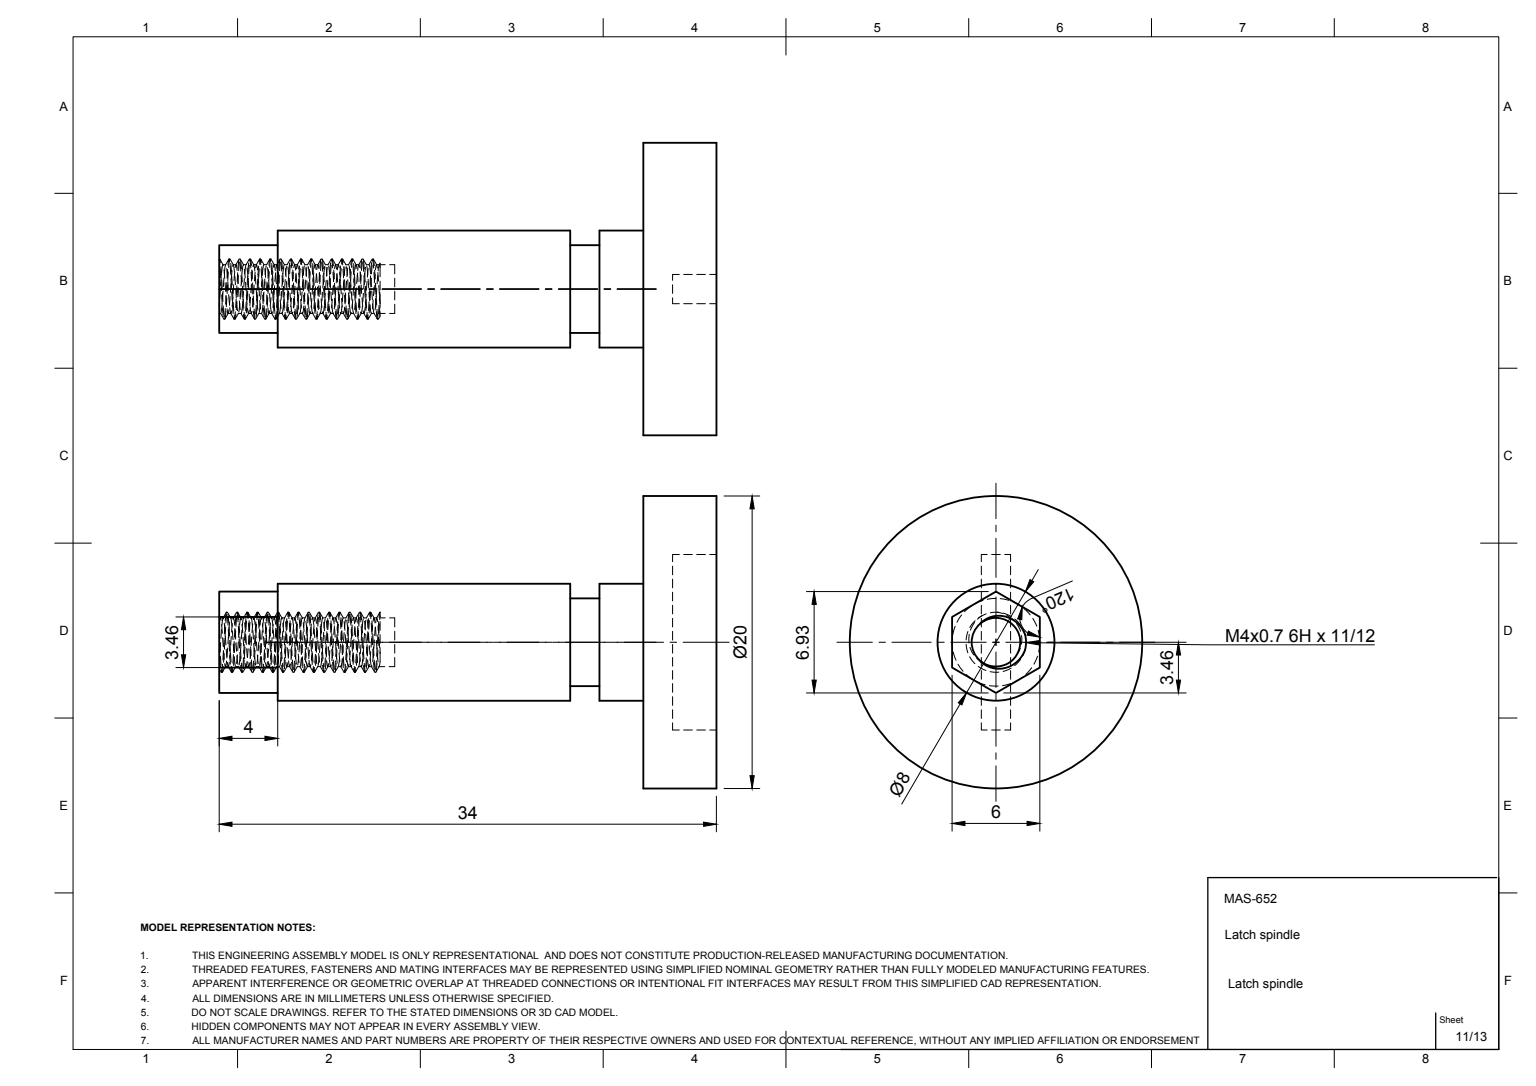
ISO-10303-21;
HEADER;
/* Generated by software containing ST-Developer
 * from STEP Tools, Inc. (www.steptools.com) 
 */

FILE_DESCRIPTION(
/* description */ ('Independent hinged machine back cover with retained hinge pins, perim
eter gasket and quarter-turn cam latch. Nominal cover 360 x 260 x 3 mm
, frame 430 x 300 x 20 mm. No guarding, structural or ingress rating a
ssigned.'),
/* implementation_level */ '2;1');

FILE_NAME(
/* name */ 'Latch spindle.step',
/* time_stamp */ '2026-11-09T19:36:59-08:00',
/* author */ (''),
/* organization */ (''),
/* preprocessor_version */ 'ST-DEVELOPER v20.2',
/* originating_system */ 'Autodesk Translation Framework v15.17.0.0',
/* authorisation */ '');

FILE_SCHEMA (('AUTOMOTIVE_DESIGN { 1 0 10303 214 3 1 1 }'));
ENDSEC;

DATA;
#10=MECHANICAL_DESIGN_GEOMETRIC_PRESENTATION_REPRESENTATION('',(#201),#32627);
#165=SHAPE_REPRESENTATION_RELATIONSHIP('SRR','None',#32711,#183);
#183=ADVANCED_BREP_SHAPE_REPRESENTATION('',(#219),#32612);
#201=STYLED_ITEM('',(#32810),#219);
#219=MANIFOLD_SOLID_BREP('Body1',#8678);
#252=FACE_BOUND('',#1180,.T.);
#253=FACE_BOUND('',#1182,.T.);
#254=FACE_BOUND('',#1191,.T.);
#255=FACE_BOUND('',#1193,.T.);
#256=FACE_BOUND('',#1196,.T.);
#257=FACE_BOUND('',#1199,.T.);
#301=B_SPLINE_SURFACE_WITH_KNOTS('',3,3,((#23063,#23064,#23065,#23066,#23067,
#23068,#23069,#23070,#23071,#23072,#23073,#23074,#23075,#23076,#23077,#23078,
#23079,#23080,#23081,#23082,#23083,#23084,#23085,#23086,#23087,#23088,#23089,
#23090,#23091,#23092,#23093,#23094,#23095,#23096,#23097,#23098,#23099,#23100,
#23101,#23102,#23103,#23104,#23105,#23106,#23107,#23108,#23109,#23110,#23111,
#23112,#23113,#23114,#23115,#23116,#23117,#23118,#23119,#23120,#23121,#23122,
#23123,#23124,#23125,#23126,#23127,#23128,#23129,#23130,#23131,#23132,#23133,
#23134,#23135,#23136,#23137,#23138,#23139,#23140,#23141,#23142,#23143,#23144,
#23145,#23146,#23147,#23148,#23149,#23150,#23151,#23152,#23153,#23154,#23155,
#23156,#23157,#23158,#23159,#23160,#23161,#23162,#23163,#23164,#23165,#23166),
(#23167,#23168,#23169,#23170,#23171,#23172,#23173,#23174,#23175,#23176,
#23177,#23178,#23179,#23180,#23181,#23182,#23183,#23184,#23185,#23186,#23187,
#23188,#23189,#23190,#23191,#23192,#23193,#23194,#23195,#23196,#23197,#23198,
#23199,#23200,#23201,#23202,#23203,#23204,#23205,#23206,#23207,#23208,#23209,
#23210,#23211,#23212,#23213,#23214,#23215,#23216,#23217,#23218,#23219,#23220,
#23221,#23222,#23223,#23224,#23225,#23226,#23227,#23228,#23229,#23230,#23231,
#23232,#23233,#23234,#23235,#23236,#23237,#23238,#23239,#23240,#23241,#23242,
#23243,#23244,#23245,#23246,#23247,#23248,#23249,#23250,#23251,#23252,#23253,
#23254,#23255,#23256,#23257,#23258,#23259,#23260,#23261,#23262,#23263,#23264,
#23265,#23266,#23267,#23268,#23269,#23270),(#23271,#23272,#23273,#23274,
#23275,#23276,#23277,#23278,#23279,#23280,#23281,#23282,#23283,#23284,#23285,
#23286,#23287,#23288,#23289,#23290,#23291,#23292,#23293,#23294,#23295,#23296,
#23297,#23298,#23299,#23300,#23301,#23302,#23303,#23304,#23305,#23306,#23307,
#23308,#23309,#23310,#23311,#23312,#23313,#23314,#23315,#23316,#23317,#23318,
#23319,#23320,#23321,#23322,#23323,#23324,#23325,#23326,#23327,#23328,#23329,
#23330,#23331,#23332,#23333,#23334,#23335,#23336,#23337,#23338,#23339,#23340,
#23341,#23342,#23343,#23344,#23345,#23346,#23347,#23348,#23349,#23350,#23351,
#23352,#23353,#23354,#23355,#23356,#23357,#23358,#23359,#23360,#23361,#23362,
#23363,#23364,#23365,#23366,#23367,#23368,#23369,#23370,#23371,#23372,#23373,
#23374),(#23375,#23376,#23377,#23378,#23379,#23380,#23381,#23382,#23383,
#23384,#23385,#23386,#23387,#23388,#23389,#23390,#23391,#23392,#23393,#23394,
#23395,#23396,#23397,#23398,#23399,#23400,#23401,#23402,#23403,#23404,#23405,
#23406,#23407,#23408,#23409,#23410,#23411,#23412,#23413,#23414,#23415,#23416,
#23417,#23418,#23419,#23420,#23421,#23422,#23423,#23424,#23425,#23426,#23427,
#23428,#23429,#23430,#23431,#23432,#23433,#23434,#23435,#23436,#23437,#23438,
#23439,#23440,#23441,#23442,#23443,#23444,#23445,#23446,#23447,#23448,#23449,
#23450,#23451,#23452,#23453,#23454,#23455,#23456,#23457,#23458,#23459,#23460,
#23461,#23462,#23463,#23464,#23465,#23466,#23467,#23468,#23469,#23470,#23471,
#23472,#23473,#23474,#23475,#23476,#23477,#23478)),.UNSPECIFIED.,.F.,.F.,
 .F.,(4,4),(4,1,1,1,1,1,1,1,1,1,1,1,1,1,1,1,1,1,1,1,1,1,1,1,1,1,1,1,1,1,
1,1,1,1,1,1,1,1,1,1,1,1,1,1,1,1,1,1,1,1,1,1,1,1,1,1,1,1,1,1,1,1,1,1,1,1,
1,1,1,1,1,1,1,1,1,1,1,1,1,1,1,1,1,1,1,1,1,1,1,1,1,1,1,1,1,1,1,1,1,1,1,4),
(0.,0.0448889834294935),(11.8615800042566,12.8591085386932,13.8566370731298,
14.8541656075664,15.851694142003,16.8492226764396,17.8467512108762,18.8442797453128,
19.8418082797494,20.839336814186,21.8368653486226,22.8343938830592,23.8319224174958,
24.8294509519324,25.826979486369,26.8245080208056,27.8220365552422,28.8195650896788,
29.8170936241154,30.814622158552,31.8121506929886,32.8096792274252,33.8072077618618,
34.8047362962984,35.802264830735,36.7997933651716,37.7973218996082,38.7948504340448,
39.7923789684814,40.789907502918,41.7874360373546,42.7849645717912,43.7824931062278,
44.7800216406644,45.777550175101,46.7750787095376,47.7726072439742,48.7701357784108,
49.7676643128474,50.765192847284,51.7627213817206,52.7602499161572,53.7577784505938,
54.7553069850304,55.752835519467,56.7503640539036,57.7478925883402,58.7454211227768,
59.7429496572134,60.74047819165,61.7380067260866,62.7355352605232,63.7330637949598,
64.7305923293964,65.728120863833,66.7256493982696,67.7231779327062,68.7207064671428,
69.7182350015794,70.715763536016,71.7132920704526,72.7108206048892,73.7083491393258,
74.7058776737624,75.703406208199,76.7009347426356,77.6984632770722,78.6959918115088,
79.6935203459454,80.691048880382,81.6885774148186,82.6861059492552,83.6836344836918,
84.6811630181284,85.678691552565,86.6762200870016,87.6737486214382,88.6712771558748,
89.6688056903114,90.666334224748,91.6638627591846,92.6613912936212,93.6589198280577,
94.6564483624943,95.6539768969309,96.6515054313676,97.6490339658042,98.6465625002407,
99.6440910346773,100.641619569114,101.639148103551,102.636676637987,103.634205172424,
104.63173370686,105.629262241297,106.626790775734,107.62431931017,108.621847844607,
109.619376379043,110.61690491348,111.614433447917,112.611961982353),
 .UNSPECIFIED.);
#302=B_SPLINE_SURFACE_WITH_KNOTS('',3,3,((#23586,#23587,#23588,#23589,#23590,
#23591,#23592,#23593,#23594,#23595,#23596,#23597,#23598,#23599,#23600,#23601,
#23602,#23603,#23604,#23605,#23606,#23607,#23608,#23609,#23610,#23611,#23612,
#23613,#23614,#23615,#23616,#23617,#23618,#23619,#23620,#23621,#23622,#23623,
#23624,#23625,#23626,#23627,#23628,#23629,#23630,#23631,#23632,#23633,#23634,
#23635,#23636,#23637,#23638,#23639,#23640,#23641,#23642,#23643,#23644,#23645,
#23646,#23647,#23648,#23649,#23650,#23651,#23652,#23653,#23654,#23655,#23656,
#23657,#23658,#23659,#23660,#23661,#23662,#23663,#23664,#23665,#23666,#23667,
#23668,#23669,#23670,#23671,#23672,#23673,#23674,#23675,#23676,#23677,#23678,
#23679,#23680,#23681,#23682,#23683,#23684,#23685,#23686,#23687,#23688,#23689),
(#23690,#23691,#23692,#23693,#23694,#23695,#23696,#23697,#23698,#23699,
#23700,#23701,#23702,#23703,#23704,#23705,#23706,#23707,#23708,#23709,#23710,
#23711,#23712,#23713,#23714,#23715,#23716,#23717,#23718,#23719,#23720,#23721,
#23722,#23723,#23724,#23725,#23726,#23727,#23728,#23729,#23730,#23731,#23732,
#23733,#23734,#23735,#23736,#23737,#23738,#23739,#23740,#23741,#23742,#23743,
#23744,#23745,#23746,#23747,#23748,#23749,#23750,#23751,#23752,#23753,#23754,
#23755,#23756,#23757,#23758,#23759,#23760,#23761,#23762,#23763,#23764,#23765,
#23766,#23767,#23768,#23769,#23770,#23771,#23772,#23773,#23774,#23775,#23776,
#23777,#23778,#23779,#23780,#23781,#23782,#23783,#23784,#23785,#23786,#23787,
#23788,#23789,#23790,#23791,#23792,#23793),(#23794,#23795,#23796,#23797,
#23798,#23799,#23800,#23801,#23802,#23803,#23804,#23805,#23806,#23807,#23808,
#23809,#23810,#23811,#23812,#23813,#23814,#23815,#23816,#23817,#23818,#23819,
#23820,#23821,#23822,#23823,#23824,#23825,#23826,#23827,#23828,#23829,#23830,
#23831,#23832,#23833,#23834,#23835,#23836,#23837,#23838,#23839,#23840,#23841,
#23842,#23843,#23844,#23845,#23846,#23847,#23848,#23849,#23850,#23851,#23852,
#23853,#23854,#23855,#23856,#23857,#23858,#23859,#23860,#23861,#23862,#23863,
#23864,#23865,#23866,#23867,#23868,#23869,#23870,#23871,#23872,#23873,#23874,
#23875,#23876,#23877,#23878,#23879,#23880,#23881,#23882,#23883,#23884,#23885,
#23886,#23887,#23888,#23889,#23890,#23891,#23892,#23893,#23894,#23895,#23896,
#23897),(#23898,#23899,#23900,#23901,#23902,#23903,#23904,#23905,#23906,
#23907,#23908,#23909,#23910,#23911,#23912,#23913,#23914,#23915,#23916,#23917,
#23918,#23919,#23920,#23921,#23922,#23923,#23924,#23925,#23926,#23927,#23928,
#23929,#23930,#23931,#23932,#23933,#23934,#23935,#23936,#23937,#23938,#23939,
#23940,#23941,#23942,#23943,#23944,#23945,#23946,#23947,#23948,#23949,#23950,
#23951,#23952,#23953,#23954,#23955,#23956,#23957,#23958,#23959,#23960,#23961,
#23962,#23963,#23964,#23965,#23966,#23967,#23968,#23969,#23970,#23971,#23972,
#23973,#23974,#23975,#23976,#23977,#23978,#23979,#23980,#23981,#23982,#23983,
#23984,#23985,#23986,#23987,#23988,#23989,#23990,#23991,#23992,#23993,#23994,
#23995,#23996,#23997,#23998,#23999,#24000,#24001)),.UNSPECIFIED.,.F.,.F.,
 .F.,(4,4),(4,1,1,1,1,1,1,1,1,1,1,1,1,1,1,1,1,1,1,1,1,1,1,1,1,1,1,1,1,1,
1,1,1,1,1,1,1,1,1,1,1,1,1,1,1,1,1,1,1,1,1,1,1,1,1,1,1,1,1,1,1,1,1,1,1,1,
1,1,1,1,1,1,1,1,1,1,1,1,1,1,1,1,1,1,1,1,1,1,1,1,1,1,1,1,1,1,1,1,1,1,1,4),
(0.,0.0448889834294935),(14.3981410127769,15.3956695472135,16.3931980816501,
17.3907266160867,18.3882551505233,19.3857836849599,20.3833122193965,21.3808407538331,
22.3783692882697,23.3758978227063,24.3734263571429,25.3709548915795,26.3684834260161,
27.3660119604527,28.3635404948893,29.3610690293259,30.3585975637625,31.3561260981991,
32.3536546326357,33.3511831670723,34.3487117015089,35.3462402359455,36.3437687703821,
37.3412973048187,38.3388258392553,39.3363543736919,40.3338829081285,41.3314114425651,
42.3289399770017,43.3264685114383,44.3239970458749,45.3215255803115,46.3190541147481,
47.3165826491847,48.3141111836213,49.3116397180579,50.3091682524945,51.3066967869311,
52.3042253213677,53.3017538558043,54.2992823902409,55.2968109246775,56.2943394591141,
57.2918679935507,58.2893965279873,59.2869250624239,60.2844535968605,61.2819821312971,
62.2795106657337,63.2770392001703,64.2745677346069,65.2720962690435,66.2696248034801,
67.2671533379167,68.2646818723533,69.2622104067898,70.2597389412265,71.2572674756631,
72.2547960100997,73.2523245445363,74.2498530789728,75.2473816134095,76.244910147846,
77.2424386822827,78.2399672167193,79.2374957511558,80.2350242855924,81.232552820029,
82.2300813544657,83.2276098889023,84.2251384233388,85.2226669577754,86.220195492212,
87.2177240266486,88.2152525610852,89.2127810955218,90.2103096299584,91.207838164395,
92.2053666988316,93.2028952332682,94.2004237677048,95.1979523021414,96.195480836578,
97.1930093710146,98.1905379054512,99.1880664398878,100.185594974324,101.183123508761,
102.180652043198,103.178180577634,104.175709112071,105.173237646507,106.170766180944,
107.168294715381,108.165823249817,109.163351784254,110.16088031869,111.158408853127,
112.155937387564,113.153465922,114.150994456437,115.148522990873),
 .UNSPECIFIED.);
#345=PLANE('',#9150);
#346=PLANE('',#9153);
#347=PLANE('',#9154);
#348=PLANE('',#9155);
#349=PLANE('',#9156);
#350=PLANE('',#9157);
#351=PLANE('',#9158);
#352=PLANE('',#9162);
#353=PLANE('',#9164);
#354=PLANE('',#9168);
#355=PLANE('',#9169);
#356=PLANE('',#9170);
#357=PLANE('',#9171);
#358=PLANE('',#9172);
#359=PLANE('',#9173);
#360=PLANE('',#9174);
#361=PLANE('',#9175);
#362=PLANE('',#9180);
#363=PLANE('',#9182);
#643=FACE_OUTER_BOUND('',#1136,.T.);
#644=FACE_OUTER_BOUND('',#1137,.T.);
#645=FACE_OUTER_BOUND('',#1138,.T.);
#646=FACE_OUTER_BOUND('',#1139,.T.);
#647=FACE_OUTER_BOUND('',#1140,.T.);
#648=FACE_OUTER_BOUND('',#1141,.T.);
#649=FACE_OUTER_BOUND('',#1142,.T.);
#650=FACE_OUTER_BOUND('',#1143,.T.);
#651=FACE_OUTER_BOUND('',#1144,.T.);
#652=FACE_OUTER_BOUND('',#1145,.T.);
#653=FACE_OUTER_BOUND('',#1146,.T.);
#654=FACE_OUTER_BOUND('',#1147,.T.);
#655=FACE_OUTER_BOUND('',#1148,.T.);
#656=FACE_OUTER_BOUND('',#1149,.T.);
#657=FACE_OUTER_BOUND('',#1150,.T.);
#658=FACE_OUTER_BOUND('',#1151,.T.);
#659=FACE_OUTER_BOUND('',#1152,.T.);
#660=FACE_OUTER_BOUND('',#1153,.T.);
#661=FACE_OUTER_BOUND('',#1154,.T.);
#662=FACE_OUTER_BOUND('',#1155,.T.);
#663=FACE_OUTER_BOUND('',#1156,.T.);
#664=FACE_OUTER_BOUND('',#1157,.T.);
#665=FACE_OUTER_BOUND('',#1158,.T.);
#666=FACE_OUTER_BOUND('',#1159,.T.);
#667=FACE_OUTER_BOUND('',#1160,.T.);
#668=FACE_OUTER_BOUND('',#1161,.T.);
#669=FACE_OUTER_BOUND('',#1162,.T.);
#670=FACE_OUTER_BOUND('',#1163,.T.);
#671=FACE_OUTER_BOUND('',#1164,.T.);
#672=FACE_OUTER_BOUND('',#1165,.T.);
#673=FACE_OUTER_BOUND('',#1166,.T.);
#674=FACE_OUTER_BOUND('',#1167,.T.);
#675=FACE_OUTER_BOUND('',#1168,.T.);
#676=FACE_OUTER_BOUND('',#1169,.T.);
#677=FACE_OUTER_BOUND('',#1170,.T.);
#678=FACE_OUTER_BOUND('',#1171,.T.);
#679=FACE_OUTER_BOUND('',#1172,.T.);
#680=FACE_OUTER_BOUND('',#1173,.T.);
#681=FACE_OUTER_BOUND('',#1174,.T.);
#682=FACE_OUTER_BOUND('',#1175,.T.);
#683=FACE_OUTER_BOUND('',#1176,.T.);
#684=FACE_OUTER_BOUND('',#1177,.T.);
#685=FACE_OUTER_BOUND('',#1178,.T.);
#686=FACE_OUTER_BOUND('',#1179,.T.);
#687=FACE_OUTER_BOUND('',#1181,.T.);
#688=FACE_OUTER_BOUND('',#1183,.T.);
#689=FACE_OUTER_BOUND('',#1184,.T.);
#690=FACE_OUTER_BOUND('',#1185,.T.);
#691=FACE_OUTER_BOUND('',#1186,.T.);
#692=FACE_OUTER_BOUND('',#1187,.T.);
#693=FACE_OUTER_BOUND('',#1188,.T.);
#694=FACE_OUTER_BOUND('',#1189,.T.);
#695=FACE_OUTER_BOUND('',#1190,.T.);
#696=FACE_OUTER_BOUND('',#1192,.T.);
#697=FACE_OUTER_BOUND('',#1194,.T.);
#698=FACE_OUTER_BOUND('',#1195,.T.);
#699=FACE_OUTER_BOUND('',#1197,.T.);
#700=FACE_OUTER_BOUND('',#1198,.T.);
#1136=EDGE_LOOP('',(#6453,#6454,#6455,#6456,#6457,#6458,#6459,#6460));
#1137=EDGE_LOOP('',(#6461,#6462,#6463,#6464));
#1138=EDGE_LOOP('',(#6465,#6466,#6467,#6468));
#1139=EDGE_LOOP('',(#6469,#6470,#6471,#6472));
#1140=EDGE_LOOP('',(#6473,#6474,#6475,#6476));
#1141=EDGE_LOOP('',(#6477,#6478,#6479,#6480));
#1142=EDGE_LOOP('',(#6481,#6482,#6483,#6484));
#1143=EDGE_LOOP('',(#6485,#6486,#6487,#6488));
#1144=EDGE_LOOP('',(#6489,#6490,#6491,#6492));
#1145=EDGE_LOOP('',(#6493,#6494,#6495,#6496));
#1146=EDGE_LOOP('',(#6497,#6498,#6499,#6500));
#1147=EDGE_LOOP('',(#6501,#6502,#6503,#6504));
#1148=EDGE_LOOP('',(#6505,#6506,#6507,#6508));
#1149=EDGE_LOOP('',(#6509,#6510,#6511,#6512));
#1150=EDGE_LOOP('',(#6513,#6514,#6515,#6516));
#1151=EDGE_LOOP('',(#6517,#6518,#6519,#6520));
#1152=EDGE_LOOP('',(#6521,#6522,#6523,#6524));
#1153=EDGE_LOOP('',(#6525,#6526,#6527,#6528));
#1154=EDGE_LOOP('',(#6529,#6530,#6531,#6532));
#1155=EDGE_LOOP('',(#6533,#6534,#6535,#6536));
#1156=EDGE_LOOP('',(#6537,#6538,#6539,#6540));
#1157=EDGE_LOOP('',(#6541,#6542,#6543,#6544));
#1158=EDGE_LOOP('',(#6545,#6546,#6547,#6548));
#1159=EDGE_LOOP('',(#6549,#6550,#6551,#6552));
#1160=EDGE_LOOP('',(#6553,#6554,#6555,#6556));
#1161=EDGE_LOOP('',(#6557,#6558,#6559,#6560));
#1162=EDGE_LOOP('',(#6561,#6562,#6563,#6564));
#1163=EDGE_LOOP('',(#6565,#6566,#6567,#6568));
#1164=EDGE_LOOP('',(#6569,#6570,#6571,#6572));
#1165=EDGE_LOOP('',(#6573,#6574,#6575,#6576));
#1166=EDGE_LOOP('',(#6577,#6578,#6579,#6580));
#1167=EDGE_LOOP('',(#6581,#6582,#6583,#6584));
#1168=EDGE_LOOP('',(#6585,#6586,#6587,#6588));
#1169=EDGE_LOOP('',(#6589,#6590,#6591,#6592,#6593,#6594,#6595,#6596,#6597,
#6598,#6599,#6600,#6601,#6602,#6603,#6604,#6605,#6606,#6607,#6608,#6609,
#6610,#6611,#6612,#6613,#6614,#6615,#6616,#6617,#6618,#6619,#6620,#6621,
#6622,#6623,#6624));
#1170=EDGE_LOOP('',(#6625,#6626,#6627,#6628,#6629,#6630,#6631,#6632,#6633,
#6634,#6635,#6636,#6637,#6638,#6639,#6640,#6641,#6642,#6643,#6644,#6645,
#6646,#6647,#6648,#6649,#6650,#6651,#6652,#6653,#6654,#6655,#6656,#6657,
#6658,#6659));
#1171=EDGE_LOOP('',(#6660,#6661,#6662,#6663));
#1172=EDGE_LOOP('',(#6664));
#1173=EDGE_LOOP('',(#6665,#6666,#6667,#6668));
#1174=EDGE_LOOP('',(#6669,#6670,#6671,#6672));
#1175=EDGE_LOOP('',(#6673,#6674,#6675,#6676));
#1176=EDGE_LOOP('',(#6677,#6678,#6679,#6680));
#1177=EDGE_LOOP('',(#6681,#6682,#6683,#6684));
#1178=EDGE_LOOP('',(#6685,#6686,#6687,#6688));
#1179=EDGE_LOOP('',(#6689));
#1180=EDGE_LOOP('',(#6690));
#1181=EDGE_LOOP('',(#6691));
#1182=EDGE_LOOP('',(#6692));
#1183=EDGE_LOOP('',(#6693,#6694,#6695,#6696));
#1184=EDGE_LOOP('',(#6697,#6698,#6699,#6700));
#1185=EDGE_LOOP('',(#6701,#6702,#6703,#6704));
#1186=EDGE_LOOP('',(#6705,#6706,#6707,#6708));
#1187=EDGE_LOOP('',(#6709,#6710,#6711,#6712));
#1188=EDGE_LOOP('',(#6713,#6714,#6715,#6716));
#1189=EDGE_LOOP('',(#6717,#6718,#6719,#6720));
#1190=EDGE_LOOP('',(#6721,#6722,#6723,#6724,#6725,#6726));
#1191=EDGE_LOOP('',(#6727,#6728,#6729,#6730));
#1192=EDGE_LOOP('',(#6731));
#1193=EDGE_LOOP('',(#6732));
#1194=EDGE_LOOP('',(#6733,#6734,#6735,#6736));
#1195=EDGE_LOOP('',(#6737));
#1196=EDGE_LOOP('',(#6738,#6739,#6740,#6741));
#1197=EDGE_LOOP('',(#6742,#6743,#6744,#6745));
#1198=EDGE_LOOP('',(#6746));
#1199=EDGE_LOOP('',(#6747,#6748,#6749,#6750,#6751,#6752));
#1495=CIRCLE('',#9115,1.666);
#1496=CIRCLE('',#9116,1.666);
#1497=CIRCLE('',#9131,1.666);
#1498=CIRCLE('',#9133,2.05475);
#1499=CIRCLE('',#9149,2.05475);
#1500=CIRCLE('',#9160,3.);
#1501=CIRCLE('',#9161,3.);
#1502=CIRCLE('',#9163,4.);
#1503=CIRCLE('',#9165,4.);
#1504=CIRCLE('',#9167,4.);
#1505=CIRCLE('',#9176,10.);
#1506=CIRCLE('',#9177,4.);
#1507=CIRCLE('',#9179,10.);
#1889=B_SPLINE_CURVE_WITH_KNOTS('',3,(#21751,#21752,#21753,#21754,#21755,
#21756,#21757,#21758,#21759,#21760,#21761,#21762,#21763,#21764,#21765,#21766,
#21767,#21768,#21769),.UNSPECIFIED.,.F.,.F.,(4,3,3,3,3,3,4),(95.5576018628658,
95.7627393059135,96.7602678403501,97.7577963747867,98.7553249092233,99.7528534436599,
100.750381978096),.UNSPECIFIED.);
#1890=B_SPLINE_CURVE_WITH_KNOTS('',3,(#21773,#21774,#21775,#21776),
 .UNSPECIFIED.,.F.,.F.,(4,4),(-98.735769112822,-98.0941628713861),
 .UNSPECIFIED.);
#1891=B_SPLINE_CURVE_WITH_KNOTS('',3,(#21780,#21781,#21782,#21783,#21784,
#21785,#21786,#21787,#21788,#21789,#21790,#21791,#21792,#21793,#21794,#21795,
#21796,#21797,#21798,#21799,#21800,#21801),.UNSPECIFIED.,.F.,.F.,(4,3,3,
3,3,3,3,4),(-98.0941628713861,-97.7577963747867,-96.7602678403501,-95.7627393059135,
-94.7652107714769,-93.7676822370403,-92.7701537026037,-91.8109775642065),
 .UNSPECIFIED.);
#1892=B_SPLINE_CURVE_WITH_KNOTS('',3,(#21806,#21807,#21808,#21809,#21810,
#21811,#21812,#21813,#21814,#21815,#21816,#21817,#21818,#21819,#21820,#21821,
#21822,#21823,#21824,#21825,#21826,#21827),.UNSPECIFIED.,.F.,.F.,(4,3,3,
3,3,3,3,4),(89.2744165556862,89.7775680992939,90.7750966337305,91.7726251681671,
92.7701537026037,93.7676822370403,94.7652107714769,95.5576018628658),
 .UNSPECIFIED.);
#1893=B_SPLINE_CURVE_WITH_KNOTS('',3,(#21828,#21829,#21830,#21831,#21832,
#21833,#21834,#21835,#21836,#21837,#21838,#21839,#21840,#21841,#21842,#21843,
#21844,#21845,#21846,#21847,#21848,#21849,#21850,#21851,#21852),
 .UNSPECIFIED.,.F.,.F.,(4,3,3,3,3,3,3,3,4),(-91.8109775642065,-91.7726251681671,
-90.7750966337305,-89.7775680992939,-88.7800395648573,-87.7825110304207,
-86.7849824959841,-85.7874539615475,-85.527792257027),.UNSPECIFIED.);
#1894=B_SPLINE_CURVE_WITH_KNOTS('',3,(#21857,#21858,#21859,#21860,#21861,
#21862,#21863,#21864,#21865,#21866,#21867,#21868,#21869,#21870,#21871,#21872,
#21873,#21874,#21875,#21876,#21877,#21878),.UNSPECIFIED.,.F.,.F.,(4,3,3,
3,3,3,3,4),(82.9912312485066,83.7923968926743,84.7899254271109,85.7874539615475,
86.7849824959841,87.7825110304207,88.7800395648573,89.2744165556862),
 .UNSPECIFIED.);
#1895=B_SPLINE_CURVE_WITH_KNOTS('',3,(#21879,#21880,#21881,#21882,#21883,
#21884,#21885,#21886,#21887,#21888,#21889,#21890,#21891,#21892,#21893,#21894,
#21895,#21896,#21897,#21898,#21899,#21900),.UNSPECIFIED.,.F.,.F.,(4,3,3,
3,3,3,3,4),(-85.527792257027,-84.7899254271109,-83.7923968926743,-82.7948683582377,
-81.7973398238011,-80.7998112893645,-79.8022827549279,-79.2446069498473),
 .UNSPECIFIED.);
#1896=B_SPLINE_CURVE_WITH_KNOTS('',3,(#21905,#21906,#21907,#21908,#21909,
#21910,#21911,#21912,#21913,#21914,#21915,#21916,#21917,#21918,#21919,#21920,
#21921,#21922,#21923,#21924,#21925,#21926,#21927,#21928,#21929),
 .UNSPECIFIED.,.F.,.F.,(4,3,3,3,3,3,3,3,4),(76.708045941327,76.8096971516181,
77.8072256860547,78.8047542204913,79.8022827549279,80.7998112893645,81.7973398238012,
82.7948683582377,82.9912312485066),.UNSPECIFIED.);
#1897=B_SPLINE_CURVE_WITH_KNOTS('',3,(#21930,#21931,#21932,#21933,#21934,
#21935,#21936,#21937,#21938,#21939,#21940,#21941,#21942,#21943,#21944,#21945,
#21946,#21947,#21948,#21949,#21950,#21951),.UNSPECIFIED.,.F.,.F.,(4,3,3,
3,3,3,3,4),(-79.2446069498473,-78.8047542204913,-77.8072256860547,-76.8096971516181,
-75.8121686171815,-74.8146400827449,-73.8171115483083,-72.9614216426677),
 .UNSPECIFIED.);
#1898=B_SPLINE_CURVE_WITH_KNOTS('',3,(#21956,#21957,#21958,#21959,#21960,
#21961,#21962,#21963,#21964,#21965,#21966,#21967,#21968,#21969,#21970,#21971,
#21972,#21973,#21974,#21975,#21976,#21977),.UNSPECIFIED.,.F.,.F.,(4,3,3,
3,3,3,3,4),(70.4248606341474,70.8245259449985,71.8220544794351,72.8195830138717,
73.8171115483083,74.8146400827449,75.8121686171815,76.708045941327),
 .UNSPECIFIED.);
#1899=B_SPLINE_CURVE_WITH_KNOTS('',3,(#21978,#21979,#21980,#21981,#21982,
#21983,#21984,#21985,#21986,#21987,#21988,#21989,#21990,#21991,#21992,#21993,
#21994,#21995,#21996,#21997,#21998,#21999,#22000,#22001,#22002),
 .UNSPECIFIED.,.F.,.F.,(4,3,3,3,3,3,3,3,4),(-72.9614216426677,-72.8195830138717,
-71.8220544794351,-70.8245259449985,-69.8269974105619,-68.8294688761253,
-67.8319403416887,-66.8344118072521,-66.6782363354882),.UNSPECIFIED.);
#1900=B_SPLINE_CURVE_WITH_KNOTS('',3,(#22007,#22008,#22009,#22010,#22011,
#22012,#22013,#22014,#22015,#22016,#22017,#22018,#22019,#22020,#22021,#22022,
#22023,#22024,#22025,#22026,#22027,#22028),.UNSPECIFIED.,.F.,.F.,(4,3,3,
3,3,3,3,4),(64.1416753269678,64.8393547383789,65.8368832728155,66.8344118072521,
67.8319403416887,68.8294688761253,69.8269974105619,70.4248606341474),
 .UNSPECIFIED.);
#1901=B_SPLINE_CURVE_WITH_KNOTS('',3,(#22029,#22030,#22031,#22032,#22033,
#22034,#22035,#22036,#22037,#22038,#22039,#22040,#22041,#22042,#22043,#22044,
#22045,#22046,#22047,#22048,#22049,#22050),.UNSPECIFIED.,.F.,.F.,(4,3,3,
3,3,3,3,4),(-66.6782363354882,-65.8368832728155,-64.8393547383789,-63.8418262039423,
-62.8442976695057,-61.8467691350691,-60.8492406006325,-60.3950510283086),
 .UNSPECIFIED.);
#1902=B_SPLINE_CURVE_WITH_KNOTS('',3,(#22055,#22056,#22057,#22058,#22059,
#22060,#22061,#22062,#22063,#22064,#22065,#22066,#22067,#22068,#22069,#22070,
#22071,#22072,#22073,#22074,#22075,#22076),.UNSPECIFIED.,.F.,.F.,(4,3,3,
3,3,3,3,4),(57.8584900197882,58.8541835317594,59.851712066196,60.8492406006326,
61.8467691350691,62.8442976695057,63.8418262039423,64.1416753269678),
 .UNSPECIFIED.);
#1903=B_SPLINE_CURVE_WITH_KNOTS('',3,(#22077,#22078,#22079,#22080,#22081,
#22082,#22083,#22084,#22085,#22086,#22087,#22088,#22089,#22090,#22091,#22092,
#22093,#22094,#22095,#22096,#22097,#22098),.UNSPECIFIED.,.F.,.F.,(4,3,3,
3,3,3,3,4),(-60.3950510283086,-59.851712066196,-58.8541835317593,-57.8566549973227,
-56.8591264628861,-55.8615979284495,-54.864069394013,-54.111865721129),
 .UNSPECIFIED.);
#1904=B_SPLINE_CURVE_WITH_KNOTS('',3,(#22103,#22104,#22105,#22106,#22107,
#22108,#22109,#22110,#22111,#22112,#22113,#22114,#22115,#22116,#22117,#22118,
#22119,#22120,#22121,#22122,#22123,#22124),.UNSPECIFIED.,.F.,.F.,(4,3,3,
3,3,3,3,4),(51.5753047126086,51.8714837907032,52.8690123251397,53.8665408595764,
54.864069394013,55.8615979284496,56.8591264628862,57.8584900197882),
 .UNSPECIFIED.);
#1905=B_SPLINE_CURVE_WITH_KNOTS('',3,(#22125,#22126,#22127,#22128,#22129,
#22130,#22131,#22132,#22133,#22134,#22135,#22136,#22137,#22138,#22139,#22140,
#22141,#22142,#22143,#22144,#22145,#22146,#22147,#22148,#22149),
 .UNSPECIFIED.,.F.,.F.,(4,3,3,3,3,3,3,3,4),(-54.111865721129,-53.8665408595764,
-52.8690123251397,-51.8714837907031,-50.8739552562666,-49.8764267218299,
-48.8788981873933,-47.8813696529567,-47.8286804139493),.UNSPECIFIED.);
#1906=B_SPLINE_CURVE_WITH_KNOTS('',3,(#22154,#22155,#22156,#22157,#22158,
#22159,#22160,#22161,#22162,#22163,#22164,#22165,#22166,#22167,#22168,#22169,
#22170,#22171,#22172,#22173,#22174,#22175),.UNSPECIFIED.,.F.,.F.,(4,3,3,
3,3,3,3,4),(45.292119405429,45.8863125840836,46.8838411185202,47.8813696529568,
48.8788981873934,49.87642672183,50.8739552562666,51.5753047126086),
 .UNSPECIFIED.);
#1907=B_SPLINE_CURVE_WITH_KNOTS('',3,(#22176,#22177,#22178,#22179,#22180,
#22181,#22182,#22183,#22184,#22185,#22186,#22187,#22188,#22189,#22190,#22191,
#22192,#22193,#22194,#22195,#22196,#22197),.UNSPECIFIED.,.F.,.F.,(4,3,3,
3,3,3,3,4),(-47.8286804139493,-46.8838411185201,-45.8863125840835,-44.888784049647,
-43.8912555152104,-42.8937269807738,-41.8961984463372,-41.5454951067698),
 .UNSPECIFIED.);
#1908=B_SPLINE_CURVE_WITH_KNOTS('',3,(#22202,#22203,#22204,#22205,#22206,
#22207,#22208,#22209,#22210,#22211,#22212,#22213,#22214,#22215,#22216,#22217,
#22218,#22219,#22220,#22221,#22222,#22223),.UNSPECIFIED.,.F.,.F.,(4,3,3,
3,3,3,3,4),(39.0089340982494,39.901141377464,40.8986699119006,41.8961984463372,
42.8937269807738,43.8912555152104,44.888784049647,45.292119405429),
 .UNSPECIFIED.);
#1909=B_SPLINE_CURVE_WITH_KNOTS('',3,(#22224,#22225,#22226,#22227,#22228,
#22229,#22230,#22231,#22232,#22233,#22234,#22235,#22236,#22237,#22238,#22239,
#22240,#22241,#22242,#22243,#22244,#22245),.UNSPECIFIED.,.F.,.F.,(4,3,3,
3,3,3,3,4),(-41.5454951067698,-40.8986699119006,-39.901141377464,-38.9036128430274,
-37.9060843085908,-36.9085557741542,-35.9110272397176,-35.2623097995902),
 .UNSPECIFIED.);
#1910=B_SPLINE_CURVE_WITH_KNOTS('',3,(#22250,#22251,#22252,#22253,#22254,
#22255,#22256,#22257,#22258,#22259,#22260,#22261,#22262,#22263,#22264,#22265,
#22266,#22267,#22268,#22269,#22270,#22271,#22272,#22273,#22274),
 .UNSPECIFIED.,.F.,.F.,(4,3,3,3,3,3,3,3,4),(32.7257487910698,32.9184416364078,
33.9159701708444,34.913498705281,35.9110272397176,36.9085557741542,37.9060843085908,
38.9036128430274,39.0089340982494),.UNSPECIFIED.);
#1911=B_SPLINE_CURVE_WITH_KNOTS('',3,(#22275,#22276,#22277,#22278,#22279,
#22280,#22281,#22282,#22283,#22284,#22285,#22286,#22287,#22288,#22289,#22290,
#22291,#22292,#22293,#22294,#22295,#22296),.UNSPECIFIED.,.F.,.F.,(4,3,3,
3,3,3,3,4),(-35.2623097995902,-34.913498705281,-33.9159701708444,-32.9184416364078,
-31.9209131019712,-30.9233845675346,-29.925856033098,-28.9791244924106),
 .UNSPECIFIED.);
#1912=B_SPLINE_CURVE_WITH_KNOTS('',3,(#22301,#22302,#22303,#22304,#22305,
#22306,#22307,#22308,#22309,#22310,#22311,#22312,#22313,#22314,#22315,#22316,
#22317,#22318,#22319,#22320,#22321,#22322),.UNSPECIFIED.,.F.,.F.,(4,3,3,
3,3,3,3,4),(26.4425634838902,26.9332704297882,27.9307989642248,28.9283274986614,
29.925856033098,30.9233845675346,31.9209131019712,32.7257487910698),
 .UNSPECIFIED.);
#1913=B_SPLINE_CURVE_WITH_KNOTS('',3,(#22323,#22324,#22325,#22326,#22327,
#22328,#22329,#22330,#22331,#22332,#22333,#22334,#22335,#22336,#22337,#22338,
#22339,#22340,#22341,#22342,#22343,#22344,#22345,#22346,#22347),
 .UNSPECIFIED.,.F.,.F.,(4,3,3,3,3,3,3,3,4),(-28.9791244924106,-28.9283274986614,
-27.9307989642248,-26.9332704297882,-25.9357418953516,-24.938213360915,
-23.9406848264784,-22.9431562920418,-22.695939185231),.UNSPECIFIED.);
#1914=B_SPLINE_CURVE_WITH_KNOTS('',3,(#22352,#22353,#22354,#22355,#22356,
#22357,#22358,#22359,#22360,#22361,#22362,#22363,#22364,#22365,#22366,#22367,
#22368,#22369,#22370,#22371,#22372,#22373),.UNSPECIFIED.,.F.,.F.,(4,3,3,
3,3,3,3,4),(20.1593781767107,20.9480992231686,21.9456277576052,22.9431562920418,
23.9406848264784,24.938213360915,25.9357418953516,26.4425634838902),
 .UNSPECIFIED.);
#1915=B_SPLINE_CURVE_WITH_KNOTS('',3,(#22374,#22375,#22376,#22377,#22378,
#22379,#22380,#22381,#22382,#22383,#22384,#22385,#22386,#22387,#22388,#22389,
#22390,#22391,#22392,#22393,#22394,#22395),.UNSPECIFIED.,.F.,.F.,(4,3,3,
3,3,3,3,4),(-22.695939185231,-21.9456277576052,-20.9480992231686,-19.950570688732,
-18.9530421542954,-17.9555136198588,-16.9579850854222,-16.4127538780514),
 .UNSPECIFIED.);
#1916=B_SPLINE_CURVE_WITH_KNOTS('',3,(#22400,#22401,#22402,#22403,#22404,
#22405,#22406,#22407,#22408,#22409,#22410,#22411,#22412,#22413,#22414,#22415,
#22416,#22417,#22418,#22419,#22420,#22421,#22422,#22423,#22424),
 .UNSPECIFIED.,.F.,.F.,(4,3,3,3,3,3,3,3,4),(13.8761928695311,13.9653994821124,
14.962928016549,15.9604565509856,16.9579850854222,17.9555136198588,18.9530421542954,
19.950570688732,20.1593781767107),.UNSPECIFIED.);
#1917=B_SPLINE_CURVE_WITH_KNOTS('',3,(#22425,#22426,#22427,#22428,#22429,
#22430,#22431,#22432,#22433,#22434,#22435,#22436,#22437,#22438,#22439,#22440,
#22441,#22442,#22443,#22444,#22445,#22446),.UNSPECIFIED.,.F.,.F.,(4,3,3,
3,3,3,3,4),(-16.4127538780514,-15.9604565509856,-14.962928016549,-13.9653994821124,
-12.9678709476758,-11.9703424132392,-10.9728138788026,-10.1295685708718),
 .UNSPECIFIED.);
#1918=B_SPLINE_CURVE_WITH_KNOTS('',3,(#22452,#22453,#22454,#22455,#22456,
#22457,#22458,#22459,#22460,#22461,#22462,#22463,#22464),.UNSPECIFIED.,
 .F.,.F.,(4,3,3,3,4),(-3.84638326369226,-2.9925856033098,-1.9950570688732,
-0.997528534436599,0.),.UNSPECIFIED.);
#1919=B_SPLINE_CURVE_WITH_KNOTS('',3,(#22467,#22468,#22469,#22470,#22471,
#22472,#22473,#22474,#22475,#22476,#22477,#22478,#22479,#22480,#22481,#22482,
#22483,#22484,#22485),.UNSPECIFIED.,.F.,.F.,(4,3,3,3,3,3,4),(2.01461286527445,
2.9925856033098,3.9901141377464,4.987642672183,5.9851712066196,6.9826997410562,
7.59300756235149),.UNSPECIFIED.);
#1920=B_SPLINE_CURVE_WITH_KNOTS('',3,(#22491,#22492,#22493,#22494,#22495,
#22496),.UNSPECIFIED.,.F.,.F.,(4,1,1,4),(109.955742875643,110.61690491348,
111.614433447917,112.611961982353),.UNSPECIFIED.);
#1921=B_SPLINE_CURVE_WITH_KNOTS('',3,(#22499,#22500,#22501,#22502,#22503,
#22504,#22505),.UNSPECIFIED.,.F.,.F.,(4,1,1,1,4),(109.955742875643,110.16088031869,
111.158408853127,112.155937387564,113.133910125599),.UNSPECIFIED.);
#1922=B_SPLINE_CURVE_WITH_KNOTS('',3,(#22510,#22511,#22512,#22513,#22514,
#22515,#22516,#22517,#22518,#22519),.UNSPECIFIED.,.F.,.F.,(4,1,1,1,1,1,
1,4),(103.672557568463,104.63173370686,105.629262241297,106.626790775734,
107.62431931017,108.621847844607,109.619376379043,109.955742875643),
 .UNSPECIFIED.);
#1923=B_SPLINE_CURVE_WITH_KNOTS('',3,(#22520,#22521,#22522,#22523,#22524,
#22525,#22526,#22527,#22528,#22529),.UNSPECIFIED.,.F.,.F.,(4,1,1,1,1,1,
1,4),(103.672557568463,104.175709112071,105.173237646507,106.170766180944,
107.168294715381,108.165823249817,109.163351784254,109.955742875643),
 .UNSPECIFIED.);
#1924=B_SPLINE_CURVE_WITH_KNOTS('',3,(#22534,#22535,#22536,#22537,#22538,
#22539,#22540,#22541,#22542,#22543,#22544),.UNSPECIFIED.,.F.,.F.,(4,1,1,
1,1,1,1,1,4),(97.3893722612836,97.6490339658042,98.6465625002407,99.6440910346773,
100.641619569114,101.639148103551,102.636676637987,103.634205172424,103.672557568463),
 .UNSPECIFIED.);
#1925=B_SPLINE_CURVE_WITH_KNOTS('',3,(#22545,#22546,#22547,#22548,#22549,
#22550,#22551,#22552,#22553,#22554),.UNSPECIFIED.,.F.,.F.,(4,1,1,1,1,1,
1,4),(97.3893722612836,98.1905379054512,99.1880664398878,100.185594974324,
101.183123508761,102.180652043198,103.178180577634,103.672557568463),
 .UNSPECIFIED.);
#1926=B_SPLINE_CURVE_WITH_KNOTS('',3,(#22559,#22560,#22561,#22562,#22563,
#22564,#22565,#22566,#22567,#22568),.UNSPECIFIED.,.F.,.F.,(4,1,1,1,1,1,
1,4),(91.106186954104,91.6638627591846,92.6613912936212,93.6589198280577,
94.6564483624943,95.6539768969309,96.6515054313676,97.3893722612836),
 .UNSPECIFIED.);
#1927=B_SPLINE_CURVE_WITH_KNOTS('',3,(#22569,#22570,#22571,#22572,#22573,
#22574,#22575,#22576,#22577,#22578,#22579),.UNSPECIFIED.,.F.,.F.,(4,1,1,
1,1,1,1,1,4),(91.106186954104,91.207838164395,92.2053666988316,93.2028952332682,
94.2004237677048,95.1979523021414,96.195480836578,97.1930093710146,97.3893722612836),
 .UNSPECIFIED.);
#1928=B_SPLINE_CURVE_WITH_KNOTS('',3,(#22584,#22585,#22586,#22587,#22588,
#22589,#22590,#22591,#22592,#22593),.UNSPECIFIED.,.F.,.F.,(4,1,1,1,1,1,
1,4),(84.8230016469244,85.678691552565,86.6762200870016,87.6737486214382,
88.6712771558748,89.6688056903114,90.666334224748,91.106186954104),
 .UNSPECIFIED.);
#1929=B_SPLINE_CURVE_WITH_KNOTS('',3,(#22594,#22595,#22596,#22597,#22598,
#22599,#22600,#22601,#22602,#22603),.UNSPECIFIED.,.F.,.F.,(4,1,1,1,1,1,
1,4),(84.8230016469244,85.2226669577754,86.220195492212,87.2177240266486,
88.2152525610852,89.2127810955218,90.2103096299584,91.106186954104),
 .UNSPECIFIED.);
#1930=B_SPLINE_CURVE_WITH_KNOTS('',3,(#22608,#22609,#22610,#22611,#22612,
#22613,#22614,#22615,#22616,#22617,#22618),.UNSPECIFIED.,.F.,.F.,(4,1,1,
1,1,1,1,1,4),(78.5398163397448,78.6959918115088,79.6935203459454,80.691048880382,
81.6885774148186,82.6861059492552,83.6836344836918,84.6811630181284,84.8230016469244),
 .UNSPECIFIED.);
#1931=B_SPLINE_CURVE_WITH_KNOTS('',3,(#22619,#22620,#22621,#22622,#22623,
#22624,#22625,#22626,#22627,#22628),.UNSPECIFIED.,.F.,.F.,(4,1,1,1,1,1,
1,4),(78.5398163397448,79.2374957511558,80.2350242855924,81.232552820029,
82.2300813544657,83.2276098889023,84.2251384233388,84.8230016469244),
 .UNSPECIFIED.);
#1932=B_SPLINE_CURVE_WITH_KNOTS('',3,(#22633,#22634,#22635,#22636,#22637,
#22638,#22639,#22640,#22641,#22642),.UNSPECIFIED.,.F.,.F.,(4,1,1,1,1,1,
1,4),(72.2566310325652,72.7108206048892,73.7083491393258,74.7058776737624,
75.703406208199,76.7009347426356,77.6984632770722,78.5398163397448),
 .UNSPECIFIED.);
#1933=B_SPLINE_CURVE_WITH_KNOTS('',3,(#22643,#22644,#22645,#22646,#22647,
#22648,#22649,#22650,#22651,#22652),.UNSPECIFIED.,.F.,.F.,(4,1,1,1,1,1,
1,4),(72.2566310325652,73.2523245445363,74.2498530789728,75.2473816134095,
76.244910147846,77.2424386822827,78.2399672167193,78.5398163397448),
 .UNSPECIFIED.);
#1934=B_SPLINE_CURVE_WITH_KNOTS('',3,(#22657,#22658,#22659,#22660,#22661,
#22662,#22663,#22664,#22665,#22666),.UNSPECIFIED.,.F.,.F.,(4,1,1,1,1,1,
1,4),(65.9734457253856,66.7256493982696,67.7231779327062,68.7207064671428,
69.7182350015794,70.715763536016,71.7132920704526,72.2566310325652),
 .UNSPECIFIED.);
#1935=B_SPLINE_CURVE_WITH_KNOTS('',3,(#22667,#22668,#22669,#22670,#22671,
#22672,#22673,#22674,#22675,#22676,#22677),.UNSPECIFIED.,.F.,.F.,(4,1,1,
1,1,1,1,1,4),(65.9734457253856,66.2696248034801,67.2671533379167,68.2646818723533,
69.2622104067898,70.2597389412265,71.2572674756631,72.2547960100997,72.2566310325652),
 .UNSPECIFIED.);
#1936=B_SPLINE_CURVE_WITH_KNOTS('',3,(#22682,#22683,#22684,#22685,#22686,
#22687,#22688,#22689,#22690,#22691,#22692),.UNSPECIFIED.,.F.,.F.,(4,1,1,
1,1,1,1,1,4),(59.690260418206,59.7429496572134,60.74047819165,61.7380067260866,
62.7355352605232,63.7330637949598,64.7305923293964,65.728120863833,65.9734457253856),
 .UNSPECIFIED.);
#1937=B_SPLINE_CURVE_WITH_KNOTS('',3,(#22693,#22694,#22695,#22696,#22697,
#22698,#22699,#22700,#22701,#22702),.UNSPECIFIED.,.F.,.F.,(4,1,1,1,1,1,
1,4),(59.690260418206,60.2844535968605,61.2819821312971,62.2795106657337,
63.2770392001703,64.2745677346069,65.2720962690435,65.9734457253856),
 .UNSPECIFIED.);
#1938=B_SPLINE_CURVE_WITH_KNOTS('',3,(#22707,#22708,#22709,#22710,#22711,
#22712,#22713,#22714,#22715,#22716),.UNSPECIFIED.,.F.,.F.,(4,1,1,1,1,1,
1,4),(53.4070751110264,53.7577784505938,54.7553069850304,55.752835519467,
56.7503640539036,57.7478925883402,58.7454211227768,59.690260418206),
 .UNSPECIFIED.);
#1939=B_SPLINE_CURVE_WITH_KNOTS('',3,(#22717,#22718,#22719,#22720,#22721,
#22722,#22723,#22724,#22725,#22726),.UNSPECIFIED.,.F.,.F.,(4,1,1,1,1,1,
1,4),(53.4070751110264,54.2992823902409,55.2968109246775,56.2943394591141,
57.2918679935507,58.2893965279873,59.2869250624239,59.690260418206),
 .UNSPECIFIED.);
#1940=B_SPLINE_CURVE_WITH_KNOTS('',3,(#22731,#22732,#22733,#22734,#22735,
#22736,#22737,#22738,#22739,#22740),.UNSPECIFIED.,.F.,.F.,(4,1,1,1,1,1,
1,4),(47.1238898038468,47.7726072439742,48.7701357784108,49.7676643128474,
50.765192847284,51.7627213817206,52.7602499161572,53.4070751110264),
 .UNSPECIFIED.);
#1941=B_SPLINE_CURVE_WITH_KNOTS('',3,(#22741,#22742,#22743,#22744,#22745,
#22746,#22747,#22748,#22749,#22750,#22751),.UNSPECIFIED.,.F.,.F.,(4,1,1,
1,1,1,1,1,4),(47.1238898038468,47.3165826491847,48.3141111836213,49.3116397180579,
50.3091682524945,51.3066967869311,52.3042253213677,53.3017538558043,53.4070751110264),
 .UNSPECIFIED.);
#1942=B_SPLINE_CURVE_WITH_KNOTS('',3,(#22756,#22757,#22758,#22759,#22760,
#22761,#22762,#22763,#22764,#22765),.UNSPECIFIED.,.F.,.F.,(4,1,1,1,1,1,
1,4),(40.8407044966673,41.7874360373546,42.7849645717912,43.7824931062278,
44.7800216406644,45.777550175101,46.7750787095376,47.1238898038468),
 .UNSPECIFIED.);
#1943=B_SPLINE_CURVE_WITH_KNOTS('',3,(#22766,#22767,#22768,#22769,#22770,
#22771,#22772,#22773,#22774,#22775),.UNSPECIFIED.,.F.,.F.,(4,1,1,1,1,1,
1,4),(40.8407044966673,41.3314114425651,42.3289399770017,43.3264685114383,
44.3239970458749,45.3215255803115,46.3190541147481,47.1238898038468),
 .UNSPECIFIED.);
#1944=B_SPLINE_CURVE_WITH_KNOTS('',3,(#22780,#22781,#22782,#22783,#22784,
#22785,#22786,#22787,#22788,#22789,#22790),.UNSPECIFIED.,.F.,.F.,(4,1,1,
1,1,1,1,1,4),(34.5575191894876,34.8047362962984,35.802264830735,36.7997933651716,
37.7973218996082,38.7948504340448,39.7923789684814,40.789907502918,40.8407044966673),
 .UNSPECIFIED.);
#1945=B_SPLINE_CURVE_WITH_KNOTS('',3,(#22791,#22792,#22793,#22794,#22795,
#22796,#22797,#22798,#22799,#22800),.UNSPECIFIED.,.F.,.F.,(4,1,1,1,1,1,
1,4),(34.5575191894876,35.3462402359455,36.3437687703821,37.3412973048187,
38.3388258392553,39.3363543736919,40.3338829081285,40.8407044966673),
 .UNSPECIFIED.);
#1946=B_SPLINE_CURVE_WITH_KNOTS('',3,(#22805,#22806,#22807,#22808,#22809,
#22810,#22811,#22812,#22813,#22814),.UNSPECIFIED.,.F.,.F.,(4,1,1,1,1,1,
1,4),(28.2743338823081,28.8195650896788,29.8170936241154,30.814622158552,
31.8121506929886,32.8096792274252,33.8072077618618,34.5575191894876),
 .UNSPECIFIED.);
#1947=B_SPLINE_CURVE_WITH_KNOTS('',3,(#22815,#22816,#22817,#22818,#22819,
#22820,#22821,#22822,#22823,#22824,#22825),.UNSPECIFIED.,.F.,.F.,(4,1,1,
1,1,1,1,1,4),(28.2743338823081,28.3635404948893,29.3610690293259,30.3585975637625,
31.3561260981991,32.3536546326357,33.3511831670723,34.3487117015089,34.5575191894876),
 .UNSPECIFIED.);
#1948=B_SPLINE_CURVE_WITH_KNOTS('',3,(#22830,#22831,#22832,#22833,#22834,
#22835,#22836,#22837,#22838,#22839),.UNSPECIFIED.,.F.,.F.,(4,1,1,1,1,1,
1,4),(21.9911485751284,22.8343938830592,23.8319224174958,24.8294509519324,
25.826979486369,26.8245080208056,27.8220365552422,28.2743338823081),
 .UNSPECIFIED.);
#1949=B_SPLINE_CURVE_WITH_KNOTS('',3,(#22840,#22841,#22842,#22843,#22844,
#22845,#22846,#22847,#22848,#22849),.UNSPECIFIED.,.F.,.F.,(4,1,1,1,1,1,
1,4),(21.9911485751284,22.3783692882697,23.3758978227063,24.3734263571429,
25.3709548915795,26.3684834260161,27.3660119604527,28.2743338823081),
 .UNSPECIFIED.);
#1950=B_SPLINE_CURVE_WITH_KNOTS('',3,(#22855,#22856,#22857,#22858,#22859),
 .UNSPECIFIED.,.F.,.F.,(4,1,4),(14.3981410127769,15.3956695472135,15.7079632679489),
 .UNSPECIFIED.);
#1951=B_SPLINE_CURVE_WITH_KNOTS('',3,(#22862,#22863,#22864,#22865,#22866),
 .UNSPECIFIED.,.F.,.F.,(4,1,4),(13.8761928695311,14.8541656075664,15.7079632679489),
 .UNSPECIFIED.);
#1952=B_SPLINE_CURVE_WITH_KNOTS('',3,(#22868,#22869,#22870,#22871,#22872,
#22873,#22874,#22875,#22876,#22877,#22878,#22879,#22880,#22881,#22882,#22883,
#22884,#22885,#22886,#22887,#22888,#22889,#22890,#22891,#22892,#22893,#22894,
#22895,#22896,#22897,#22898,#22899,#22900,#22901,#22902,#22903,#22904,#22905,
#22906,#22907,#22908,#22909,#22910,#22911,#22912,#22913,#22914,#22915,#22916,
#22917,#22918,#22919,#22920,#22921,#22922,#22923,#22924,#22925,#22926,#22927,
#22928,#22929,#22930,#22931,#22932,#22933,#22934,#22935,#22936,#22937,#22938,
#22939,#22940,#22941,#22942,#22943,#22944,#22945,#22946,#22947,#22948,#22949,
#22950,#22951,#22952,#22953,#22954,#22955),.UNSPECIFIED.,.F.,.F.,(4,3,3,
3,3,3,3,3,3,3,3,3,3,3,3,3,3,3,3,3,3,3,3,3,3,3,3,3,3,4),(-0.378621596831403,
-0.359793800533641,-0.347850189670991,-0.339636048942975,-0.335335774136304,
-0.31546051317345,-0.301132643095686,-0.297156907494375,-0.293211954051928,
-0.272807042011262,-0.252109806400788,-0.239291742938424,-0.228786234997388,
-0.224498858881779,-0.203194502850499,-0.200837552551333,-0.180352825937995,
-0.158313007596234,-0.154345292986098,-0.150812110310244,-0.129430920910395,
-0.107597661495996,-0.0856310553157248,-0.0802130557452004,-0.0759476002900926,
-0.0534004481199611,-0.0308282090279777,-0.00877005394723412,-0.00403427920391026,
0.),.UNSPECIFIED.);
#1953=B_SPLINE_CURVE_WITH_KNOTS('',3,(#22956,#22957,#22958,#22959,#22960,
#22961,#22962,#22963,#22964,#22965,#22966,#22967,#22968,#22969,#22970,#22971,
#22972,#22973,#22974,#22975,#22976,#22977,#22978,#22979,#22980,#22981,#22982,
#22983,#22984,#22985,#22986,#22987,#22988,#22989,#22990,#22991,#22992,#22993,
#22994,#22995,#22996,#22997,#22998,#22999,#23000,#23001,#23002,#23003,#23004,
#23005,#23006,#23007,#23008,#23009,#23010,#23011,#23012,#23013,#23014,#23015,
#23016,#23017,#23018,#23019,#23020,#23021,#23022,#23023,#23024,#23025,#23026,
#23027,#23028,#23029,#23030,#23031,#23032,#23033,#23034,#23035,#23036,#23037,
#23038,#23039,#23040),.UNSPECIFIED.,.F.,.F.,(4,3,3,3,3,3,3,3,3,3,3,3,3,
3,3,3,3,3,3,3,3,3,3,3,3,3,3,3,4),(-0.376940817211647,-0.354631959429703,
-0.332910822711019,-0.32806220569962,-0.305813663335352,-0.290194813628462,
-0.284256552410819,-0.278600734522432,-0.256917979000876,-0.235701442818543,
-0.214949892844509,-0.208195692337994,-0.204402258299287,-0.183827120255531,
-0.180862865680235,-0.159880225304417,-0.140305799915047,-0.136023059343962,
-0.132589312410188,-0.11212985906865,-0.0917656064462646,-0.0718387373507178,
-0.0676299187791264,-0.0636628529112296,-0.044105741114238,-0.024921443999485,
-0.00636112761058051,-0.00328482218945467,0.),.UNSPECIFIED.);
#1954=B_SPLINE_CURVE_WITH_KNOTS('',3,(#23042,#23043,#23044,#23045,#23046,
#23047,#23048,#23049,#23050,#23051,#23052),.UNSPECIFIED.,.F.,.F.,(4,1,1,
1,1,1,1,1,4),(15.7079632679489,15.851694142003,16.8492226764396,17.8467512108762,
18.8442797453128,19.8418082797494,20.839336814186,21.8368653486226,21.9911485751284),
 .UNSPECIFIED.);
#1955=B_SPLINE_CURVE_WITH_KNOTS('',3,(#23053,#23054,#23055,#23056,#23057,
#23058,#23059,#23060,#23061,#23062),.UNSPECIFIED.,.F.,.F.,(4,1,1,1,1,1,
1,4),(15.7079632679489,16.3931980816501,17.3907266160867,18.3882551505233,
19.3857836849599,20.3833122193965,21.3808407538331,21.9911485751284),
 .UNSPECIFIED.);
#1956=B_SPLINE_CURVE_WITH_KNOTS('',3,(#23479,#23480,#23481,#23482,#23483,
#23484,#23485,#23486,#23487,#23488,#23489,#23490,#23491,#23492,#23493,#23494,
#23495,#23496,#23497,#23498,#23499,#23500,#23501,#23502,#23503,#23504,#23505,
#23506,#23507,#23508,#23509,#23510,#23511,#23512,#23513,#23514,#23515,#23516,
#23517,#23518,#23519,#23520,#23521,#23522,#23523,#23524,#23525,#23526,#23527,
#23528,#23529,#23530,#23531,#23532,#23533,#23534,#23535,#23536,#23537,#23538,
#23539,#23540,#23541,#23542,#23543,#23544,#23545,#23546,#23547,#23548,#23549,
#23550,#23551,#23552,#23553,#23554,#23555,#23556,#23557,#23558,#23559,#23560),
 .UNSPECIFIED.,.F.,.F.,(4,3,3,3,3,3,3,3,3,3,3,3,3,3,3,3,3,3,3,3,3,3,3,3,
3,3,3,4),(0.,0.0186013309220082,0.0384258187432639,0.0557722455868627,0.064476526623233,
0.0684519336897636,0.0885088376090689,0.108919913995898,0.125989243869937,
0.133854361750648,0.137287827509053,0.158362305677327,0.177197233492054,
0.197723029954501,0.205648563033172,0.209124559961607,0.230127910462039,
0.251618950585589,0.268076130837863,0.278319720735245,0.284044100051126,
0.30631294997178,0.322965504893635,0.328171461506484,0.333183430590058,
0.355704845535606,0.372923169659198,0.376940817211655),.UNSPECIFIED.);
#1957=B_SPLINE_CURVE_WITH_KNOTS('',3,(#23561,#23562,#23563,#23564,#23565,
#23566,#23567,#23568,#23569,#23570,#23571,#23572,#23573,#23574,#23575,#23576,
#23577,#23578,#23579,#23580,#23581,#23582,#23583,#23584,#23585),
 .UNSPECIFIED.,.F.,.F.,(4,3,3,3,3,3,3,3,4),(-10.1295685708718,-9.97528534436599,
-8.97775680992939,-7.98022827549279,-6.98269974105619,-5.98517120661959,
-4.98764267218299,-3.9901141377464,-3.84638326369226),.UNSPECIFIED.);
#1958=B_SPLINE_CURVE_WITH_KNOTS('',3,(#24002,#24003,#24004,#24005,#24006,
#24007,#24008,#24009,#24010,#24011,#24012,#24013,#24014,#24015,#24016,#24017,
#24018,#24019,#24020,#24021,#24022,#24023),.UNSPECIFIED.,.F.,.F.,(4,3,3,
3,3,3,3,4),(7.59300756235149,7.98022827549279,8.97775680992939,9.97528534436599,
10.9728138788026,11.9703424132392,12.9678709476758,13.8761928695311),
 .UNSPECIFIED.);
#1959=B_SPLINE_CURVE_WITH_KNOTS('',3,(#24024,#24025,#24026,#24027,#24028,
#24029,#24030,#24031,#24032,#24033,#24034,#24035,#24036,#24037,#24038,#24039,
#24040,#24041,#24042,#24043,#24044,#24045,#24046,#24047,#24048,#24049,#24050,
#24051,#24052,#24053,#24054,#24055,#24056,#24057,#24058,#24059,#24060,#24061,
#24062,#24063,#24064,#24065,#24066,#24067,#24068,#24069,#24070,#24071,#24072,
#24073,#24074,#24075,#24076,#24077,#24078,#24079,#24080,#24081,#24082,#24083,
#24084,#24085,#24086,#24087,#24088,#24089,#24090,#24091,#24092,#24093,#24094,
#24095,#24096,#24097,#24098,#24099,#24100,#24101,#24102,#24103,#24104,#24105,
#24106,#24107,#24108),.UNSPECIFIED.,.F.,.F.,(4,3,3,3,3,3,3,3,3,3,3,3,3,
3,3,3,3,3,3,3,3,3,3,3,3,3,3,3,4),(0.,0.0219693271129621,0.0445470856655639,
0.0636231399133006,0.0720978574378349,0.0767563405636669,0.0810490577745036,
0.102995570811128,0.124770875307109,0.142867036392196,0.150422875677093,
0.153918682854505,0.157566935291381,0.178336708531301,0.197155519647457,
0.219426672701596,0.224327949631498,0.229401226278881,0.250066427413625,
0.27072708362855,0.285673099166475,0.296886737298637,0.300621606934625,
0.320392720001204,0.334297633865279,0.338764463536532,0.35778760385162,
0.375324744080566,0.378621596831418),.UNSPECIFIED.);
#2380=LINE('',#21749,#2926);
#2381=LINE('',#21778,#2927);
#2382=LINE('',#21805,#2928);
#2383=LINE('',#21856,#2929);
#2384=LINE('',#21904,#2930);
#2385=LINE('',#21955,#2931);
#2386=LINE('',#22006,#2932);
#2387=LINE('',#22054,#2933);
#2388=LINE('',#22102,#2934);
#2389=LINE('',#22153,#2935);
#2390=LINE('',#22201,#2936);
#2391=LINE('',#22249,#2937);
#2392=LINE('',#22300,#2938);
#2393=LINE('',#22351,#2939);
#2394=LINE('',#22399,#2940);
#2395=LINE('',#22450,#2941);
#2396=LINE('',#22489,#2942);
#2397=LINE('',#22509,#2943);
#2398=LINE('',#22533,#2944);
#2399=LINE('',#22558,#2945);
#2400=LINE('',#22583,#2946);
#2401=LINE('',#22607,#2947);
#2402=LINE('',#22632,#2948);
#2403=LINE('',#22656,#2949);
#2404=LINE('',#22681,#2950);
#2405=LINE('',#22706,#2951);
#2406=LINE('',#22730,#2952);
#2407=LINE('',#22755,#2953);
#2408=LINE('',#22779,#2954);
#2409=LINE('',#22804,#2955);
#2410=LINE('',#22829,#2956);
#2411=LINE('',#22853,#2957);
#2412=LINE('',#24114,#2958);
#2413=LINE('',#24116,#2959);
#2414=LINE('',#24118,#2960);
#2415=LINE('',#24119,#2961);
#2416=LINE('',#24122,#2962);
#2417=LINE('',#24124,#2963);
#2418=LINE('',#24125,#2964);
#2419=LINE('',#24128,#2965);
#2420=LINE('',#24130,#2966);
#2421=LINE('',#24131,#2967);
#2422=LINE('',#24133,#2968);
#2423=LINE('',#24134,#2969);
#2424=LINE('',#24140,#2970);
#2425=LINE('',#24151,#2971);
#2426=LINE('',#24155,#2972);
#2427=LINE('',#24157,#2973);
#2428=LINE('',#24159,#2974);
#2429=LINE('',#24160,#2975);
#2430=LINE('',#24163,#2976);
#2431=LINE('',#24165,#2977);
#2432=LINE('',#24166,#2978);
#2433=LINE('',#24169,#2979);
#2434=LINE('',#24171,#2980);
#2435=LINE('',#24172,#2981);
#2436=LINE('',#24175,#2982);
#2437=LINE('',#24177,#2983);
#2438=LINE('',#24178,#2984);
#2439=LINE('',#24181,#2985);
#2440=LINE('',#24183,#2986);
#2441=LINE('',#24184,#2987);
#2442=LINE('',#24186,#2988);
#2443=LINE('',#24187,#2989);
#2444=LINE('',#24196,#2990);
#2445=LINE('',#24200,#2991);
#2926=VECTOR('',#10180,2.);
#2927=VECTOR('',#10183,2.);
#2928=VECTOR('',#10188,2.);
#2929=VECTOR('',#10191,2.);
#2930=VECTOR('',#10194,2.);
#2931=VECTOR('',#10197,2.);
#2932=VECTOR('',#10200,2.);
#2933=VECTOR('',#10203,2.);
#2934=VECTOR('',#10206,2.);
#2935=VECTOR('',#10209,2.);
#2936=VECTOR('',#10212,2.);
#2937=VECTOR('',#10215,2.);
#2938=VECTOR('',#10218,2.);
#2939=VECTOR('',#10221,2.);
#2940=VECTOR('',#10224,2.);
#2941=VECTOR('',#10227,2.);
#2942=VECTOR('',#10232,2.05475);
#2943=VECTOR('',#10237,2.05475);
#2944=VECTOR('',#10240,2.05475);
#2945=VECTOR('',#10243,2.05475);
#2946=VECTOR('',#10246,2.05475);
#2947=VECTOR('',#10249,2.05475);
#2948=VECTOR('',#10252,2.05475);
#2949=VECTOR('',#10255,2.05475);
#2950=VECTOR('',#10258,2.05475);
#2951=VECTOR('',#10261,2.05475);
#2952=VECTOR('',#10264,2.05475);
#2953=VECTOR('',#10267,2.05475);
#2954=VECTOR('',#10270,2.05475);
#2955=VECTOR('',#10273,2.05475);
#2956=VECTOR('',#10276,2.05475);
#2957=VECTOR('',#10279,2.05475);
#2958=VECTOR('',#10292,10.);
#2959=VECTOR('',#10293,10.);
#2960=VECTOR('',#10294,10.);
#2961=VECTOR('',#10295,10.);
#2962=VECTOR('',#10298,10.);
#2963=VECTOR('',#10299,10.);
#2964=VECTOR('',#10300,10.);
#2965=VECTOR('',#10303,10.);
#2966=VECTOR('',#10304,10.);
#2967=VECTOR('',#10305,10.);
#2968=VECTOR('',#10308,10.);
#2969=VECTOR('',#10309,10.);
#2970=VECTOR('',#10316,3.);
#2971=VECTOR('',#10331,4.);
#2972=VECTOR('',#10334,10.);
#2973=VECTOR('',#10335,10.);
#2974=VECTOR('',#10336,10.);
#2975=VECTOR('',#10337,10.);
#2976=VECTOR('',#10340,10.);
#2977=VECTOR('',#10341,10.);
#2978=VECTOR('',#10342,10.);
#2979=VECTOR('',#10345,10.);
#2980=VECTOR('',#10346,10.);
#2981=VECTOR('',#10347,10.);
#2982=VECTOR('',#10350,10.);
#2983=VECTOR('',#10351,10.);
#2984=VECTOR('',#10352,10.);
#2985=VECTOR('',#10355,10.);
#2986=VECTOR('',#10356,10.);
#2987=VECTOR('',#10357,10.);
#2988=VECTOR('',#10360,10.);
#2989=VECTOR('',#10361,10.);
#2990=VECTOR('',#10372,10.);
#2991=VECTOR('',#10379,4.);
#3629=VERTEX_POINT('',#21747);
#3630=VERTEX_POINT('',#21748);
#3631=VERTEX_POINT('',#21750);
#3632=VERTEX_POINT('',#21770);
#3633=VERTEX_POINT('',#21772);
#3634=VERTEX_POINT('',#21777);
#3635=VERTEX_POINT('',#21803);
#3636=VERTEX_POINT('',#21804);
#3637=VERTEX_POINT('',#21854);
#3638=VERTEX_POINT('',#21855);
#3639=VERTEX_POINT('',#21902);
#3640=VERTEX_POINT('',#21903);
#3641=VERTEX_POINT('',#21953);
#3642=VERTEX_POINT('',#21954);
#3643=VERTEX_POINT('',#22004);
#3644=VERTEX_POINT('',#22005);
#3645=VERTEX_POINT('',#22052);
#3646=VERTEX_POINT('',#22053);
#3647=VERTEX_POINT('',#22100);
#3648=VERTEX_POINT('',#22101);
#3649=VERTEX_POINT('',#22151);
#3650=VERTEX_POINT('',#22152);
#3651=VERTEX_POINT('',#22199);
#3652=VERTEX_POINT('',#22200);
#3653=VERTEX_POINT('',#22247);
#3654=VERTEX_POINT('',#22248);
#3655=VERTEX_POINT('',#22298);
#3656=VERTEX_POINT('',#22299);
#3657=VERTEX_POINT('',#22349);
#3658=VERTEX_POINT('',#22350);
#3659=VERTEX_POINT('',#22397);
#3660=VERTEX_POINT('',#22398);
#3661=VERTEX_POINT('',#22448);
#3662=VERTEX_POINT('',#22449);
#3663=VERTEX_POINT('',#22451);
#3664=VERTEX_POINT('',#22465);
#3665=VERTEX_POINT('',#22487);
#3666=VERTEX_POINT('',#22488);
#3667=VERTEX_POINT('',#22490);
#3668=VERTEX_POINT('',#22497);
#3669=VERTEX_POINT('',#22507);
#3670=VERTEX_POINT('',#22508);
#3671=VERTEX_POINT('',#22531);
#3672=VERTEX_POINT('',#22532);
#3673=VERTEX_POINT('',#22556);
#3674=VERTEX_POINT('',#22557);
#3675=VERTEX_POINT('',#22581);
#3676=VERTEX_POINT('',#22582);
#3677=VERTEX_POINT('',#22605);
#3678=VERTEX_POINT('',#22606);
#3679=VERTEX_POINT('',#22630);
#3680=VERTEX_POINT('',#22631);
#3681=VERTEX_POINT('',#22654);
#3682=VERTEX_POINT('',#22655);
#3683=VERTEX_POINT('',#22679);
#3684=VERTEX_POINT('',#22680);
#3685=VERTEX_POINT('',#22704);
#3686=VERTEX_POINT('',#22705);
#3687=VERTEX_POINT('',#22728);
#3688=VERTEX_POINT('',#22729);
#3689=VERTEX_POINT('',#22753);
#3690=VERTEX_POINT('',#22754);
#3691=VERTEX_POINT('',#22777);
#3692=VERTEX_POINT('',#22778);
#3693=VERTEX_POINT('',#22802);
#3694=VERTEX_POINT('',#22803);
#3695=VERTEX_POINT('',#22827);
#3696=VERTEX_POINT('',#22828);
#3697=VERTEX_POINT('',#22851);
#3698=VERTEX_POINT('',#22852);
#3699=VERTEX_POINT('',#22854);
#3700=VERTEX_POINT('',#22860);
#3701=VERTEX_POINT('',#24112);
#3702=VERTEX_POINT('',#24113);
#3703=VERTEX_POINT('',#24115);
#3704=VERTEX_POINT('',#24117);
#3705=VERTEX_POINT('',#24121);
#3706=VERTEX_POINT('',#24123);
#3707=VERTEX_POINT('',#24127);
#3708=VERTEX_POINT('',#24129);
#3709=VERTEX_POINT('',#24137);
#3710=VERTEX_POINT('',#24139);
#3711=VERTEX_POINT('',#24143);
#3712=VERTEX_POINT('',#24146);
#3713=VERTEX_POINT('',#24149);
#3714=VERTEX_POINT('',#24153);
#3715=VERTEX_POINT('',#24154);
#3716=VERTEX_POINT('',#24156);
#3717=VERTEX_POINT('',#24158);
#3718=VERTEX_POINT('',#24162);
#3719=VERTEX_POINT('',#24164);
#3720=VERTEX_POINT('',#24168);
#3721=VERTEX_POINT('',#24170);
#3722=VERTEX_POINT('',#24174);
#3723=VERTEX_POINT('',#24176);
#3724=VERTEX_POINT('',#24180);
#3725=VERTEX_POINT('',#24182);
#3726=VERTEX_POINT('',#24190);
#3727=VERTEX_POINT('',#24192);
#3728=VERTEX_POINT('',#24195);
#4650=EDGE_CURVE('',#3629,#3630,#2380,.T.);
#4651=EDGE_CURVE('',#3630,#3631,#1889,.T.);
#4652=EDGE_CURVE('',#3631,#3632,#1495,.T.);
#4653=EDGE_CURVE('',#3632,#3633,#1890,.T.);
#4654=EDGE_CURVE('',#3633,#3634,#2381,.T.);
#4655=EDGE_CURVE('',#3634,#3634,#1496,.F.);
#4656=EDGE_CURVE('',#3633,#3629,#1891,.T.);
#4657=EDGE_CURVE('',#3635,#3636,#2382,.T.);
#4658=EDGE_CURVE('',#3636,#3630,#1892,.T.);
#4659=EDGE_CURVE('',#3629,#3635,#1893,.T.);
#4660=EDGE_CURVE('',#3637,#3638,#2383,.T.);
#4661=EDGE_CURVE('',#3638,#3636,#1894,.T.);
#4662=EDGE_CURVE('',#3635,#3637,#1895,.T.);
#4663=EDGE_CURVE('',#3639,#3640,#2384,.T.);
#4664=EDGE_CURVE('',#3640,#3638,#1896,.T.);
#4665=EDGE_CURVE('',#3637,#3639,#1897,.T.);
#4666=EDGE_CURVE('',#3641,#3642,#2385,.T.);
#4667=EDGE_CURVE('',#3642,#3640,#1898,.T.);
#4668=EDGE_CURVE('',#3639,#3641,#1899,.T.);
#4669=EDGE_CURVE('',#3643,#3644,#2386,.T.);
#4670=EDGE_CURVE('',#3644,#3642,#1900,.T.);
#4671=EDGE_CURVE('',#3641,#3643,#1901,.T.);
#4672=EDGE_CURVE('',#3645,#3646,#2387,.T.);
#4673=EDGE_CURVE('',#3646,#3644,#1902,.T.);
#4674=EDGE_CURVE('',#3643,#3645,#1903,.T.);
#4675=EDGE_CURVE('',#3647,#3648,#2388,.T.);
#4676=EDGE_CURVE('',#3648,#3646,#1904,.T.);
#4677=EDGE_CURVE('',#3645,#3647,#1905,.T.);
#4678=EDGE_CURVE('',#3649,#3650,#2389,.T.);
#4679=EDGE_CURVE('',#3650,#3648,#1906,.T.);
#4680=EDGE_CURVE('',#3647,#3649,#1907,.T.);
#4681=EDGE_CURVE('',#3651,#3652,#2390,.T.);
#4682=EDGE_CURVE('',#3652,#3650,#1908,.T.);
#4683=EDGE_CURVE('',#3649,#3651,#1909,.T.);
#4684=EDGE_CURVE('',#3653,#3654,#2391,.T.);
#4685=EDGE_CURVE('',#3654,#3652,#1910,.T.);
#4686=EDGE_CURVE('',#3651,#3653,#1911,.T.);
#4687=EDGE_CURVE('',#3655,#3656,#2392,.T.);
#4688=EDGE_CURVE('',#3656,#3654,#1912,.T.);
#4689=EDGE_CURVE('',#3653,#3655,#1913,.T.);
#4690=EDGE_CURVE('',#3657,#3658,#2393,.T.);
#4691=EDGE_CURVE('',#3658,#3656,#1914,.T.);
#4692=EDGE_CURVE('',#3655,#3657,#1915,.T.);
#4693=EDGE_CURVE('',#3659,#3660,#2394,.T.);
#4694=EDGE_CURVE('',#3660,#3658,#1916,.T.);
#4695=EDGE_CURVE('',#3657,#3659,#1917,.T.);
#4696=EDGE_CURVE('',#3661,#3662,#2395,.T.);
#4697=EDGE_CURVE('',#3661,#3663,#1918,.T.);
#4698=EDGE_CURVE('',#3664,#3663,#1497,.T.);
#4699=EDGE_CURVE('',#3664,#3662,#1919,.T.);
#4700=EDGE_CURVE('',#3665,#3666,#2396,.T.);
#4701=EDGE_CURVE('',#3666,#3667,#1920,.T.);
#4702=EDGE_CURVE('',#3668,#3667,#1498,.T.);
#4703=EDGE_CURVE('',#3665,#3668,#1921,.T.);
#4704=EDGE_CURVE('',#3669,#3670,#2397,.T.);
#4705=EDGE_CURVE('',#3670,#3666,#1922,.T.);
#4706=EDGE_CURVE('',#3669,#3665,#1923,.T.);
#4707=EDGE_CURVE('',#3671,#3672,#2398,.T.);
#4708=EDGE_CURVE('',#3672,#3670,#1924,.T.);
#4709=EDGE_CURVE('',#3671,#3669,#1925,.T.);
#4710=EDGE_CURVE('',#3673,#3674,#2399,.T.);
#4711=EDGE_CURVE('',#3674,#3672,#1926,.T.);
#4712=EDGE_CURVE('',#3673,#3671,#1927,.T.);
#4713=EDGE_CURVE('',#3675,#3676,#2400,.T.);
#4714=EDGE_CURVE('',#3676,#3674,#1928,.T.);
#4715=EDGE_CURVE('',#3675,#3673,#1929,.T.);
#4716=EDGE_CURVE('',#3677,#3678,#2401,.T.);
#4717=EDGE_CURVE('',#3678,#3676,#1930,.T.);
#4718=EDGE_CURVE('',#3677,#3675,#1931,.T.);
#4719=EDGE_CURVE('',#3679,#3680,#2402,.T.);
#4720=EDGE_CURVE('',#3680,#3678,#1932,.T.);
#4721=EDGE_CURVE('',#3679,#3677,#1933,.T.);
#4722=EDGE_CURVE('',#3681,#3682,#2403,.T.);
#4723=EDGE_CURVE('',#3682,#3680,#1934,.T.);
#4724=EDGE_CURVE('',#3681,#3679,#1935,.T.);
#4725=EDGE_CURVE('',#3683,#3684,#2404,.T.);
#4726=EDGE_CURVE('',#3684,#3682,#1936,.T.);
#4727=EDGE_CURVE('',#3683,#3681,#1937,.T.);
#4728=EDGE_CURVE('',#3685,#3686,#2405,.T.);
#4729=EDGE_CURVE('',#3686,#3684,#1938,.T.);
#4730=EDGE_CURVE('',#3685,#3683,#1939,.T.);
#4731=EDGE_CURVE('',#3687,#3688,#2406,.T.);
#4732=EDGE_CURVE('',#3688,#3686,#1940,.T.);
#4733=EDGE_CURVE('',#3687,#3685,#1941,.T.);
#4734=EDGE_CURVE('',#3689,#3690,#2407,.T.);
#4735=EDGE_CURVE('',#3690,#3688,#1942,.T.);
#4736=EDGE_CURVE('',#3689,#3687,#1943,.T.);
#4737=EDGE_CURVE('',#3691,#3692,#2408,.T.);
#4738=EDGE_CURVE('',#3692,#3690,#1944,.T.);
#4739=EDGE_CURVE('',#3691,#3689,#1945,.T.);
#4740=EDGE_CURVE('',#3693,#3694,#2409,.T.);
#4741=EDGE_CURVE('',#3694,#3692,#1946,.T.);
#4742=EDGE_CURVE('',#3693,#3691,#1947,.T.);
#4743=EDGE_CURVE('',#3695,#3696,#2410,.T.);
#4744=EDGE_CURVE('',#3696,#3694,#1948,.T.);
#4745=EDGE_CURVE('',#3695,#3693,#1949,.T.);
#4746=EDGE_CURVE('',#3697,#3698,#2411,.T.);
#4747=EDGE_CURVE('',#3699,#3697,#1950,.T.);
#4748=EDGE_CURVE('',#3700,#3699,#1499,.T.);
#4749=EDGE_CURVE('',#3700,#3698,#1951,.T.);
#4750=EDGE_CURVE('',#3631,#3668,#1952,.T.);
#4751=EDGE_CURVE('',#3667,#3632,#1953,.T.);
#4752=EDGE_CURVE('',#3698,#3696,#1954,.T.);
#4753=EDGE_CURVE('',#3697,#3695,#1955,.T.);
#4754=EDGE_CURVE('',#3663,#3700,#1956,.T.);
#4755=EDGE_CURVE('',#3659,#3661,#1957,.T.);
#4756=EDGE_CURVE('',#3662,#3660,#1958,.T.);
#4757=EDGE_CURVE('',#3699,#3664,#1959,.T.);
#4758=EDGE_CURVE('',#3701,#3702,#2412,.T.);
#4759=EDGE_CURVE('',#3702,#3703,#2413,.T.);
#4760=EDGE_CURVE('',#3704,#3703,#2414,.T.);
#4761=EDGE_CURVE('',#3701,#3704,#2415,.T.);
#4762=EDGE_CURVE('',#3702,#3705,#2416,.T.);
#4763=EDGE_CURVE('',#3705,#3706,#2417,.T.);
#4764=EDGE_CURVE('',#3703,#3706,#2418,.T.);
#4765=EDGE_CURVE('',#3705,#3707,#2419,.T.);
#4766=EDGE_CURVE('',#3707,#3708,#2420,.T.);
#4767=EDGE_CURVE('',#3706,#3708,#2421,.T.);
#4768=EDGE_CURVE('',#3707,#3701,#2422,.T.);
#4769=EDGE_CURVE('',#3708,#3704,#2423,.T.);
#4770=EDGE_CURVE('',#3709,#3709,#1500,.T.);
#4771=EDGE_CURVE('',#3709,#3710,#2424,.T.);
#4772=EDGE_CURVE('',#3710,#3710,#1501,.T.);
#4773=EDGE_CURVE('',#3711,#3711,#1502,.T.);
#4774=EDGE_CURVE('',#3712,#3712,#1503,.T.);
#4775=EDGE_CURVE('',#3713,#3713,#1504,.T.);
#4776=EDGE_CURVE('',#3713,#3712,#2425,.T.);
#4777=EDGE_CURVE('',#3714,#3715,#2426,.T.);
#4778=EDGE_CURVE('',#3714,#3716,#2427,.T.);
#4779=EDGE_CURVE('',#3717,#3716,#2428,.T.);
#4780=EDGE_CURVE('',#3715,#3717,#2429,.T.);
#4781=EDGE_CURVE('',#3715,#3718,#2430,.T.);
#4782=EDGE_CURVE('',#3719,#3717,#2431,.T.);
#4783=EDGE_CURVE('',#3718,#3719,#2432,.T.);
#4784=EDGE_CURVE('',#3718,#3720,#2433,.T.);
#4785=EDGE_CURVE('',#3721,#3719,#2434,.T.);
#4786=EDGE_CURVE('',#3720,#3721,#2435,.T.);
#4787=EDGE_CURVE('',#3720,#3722,#2436,.T.);
#4788=EDGE_CURVE('',#3723,#3721,#2437,.T.);
#4789=EDGE_CURVE('',#3722,#3723,#2438,.T.);
#4790=EDGE_CURVE('',#3722,#3724,#2439,.T.);
#4791=EDGE_CURVE('',#3725,#3723,#2440,.T.);
#4792=EDGE_CURVE('',#3724,#3725,#2441,.T.);
#4793=EDGE_CURVE('',#3724,#3714,#2442,.T.);
#4794=EDGE_CURVE('',#3716,#3725,#2443,.T.);
#4795=EDGE_CURVE('',#3726,#3726,#1505,.T.);
#4796=EDGE_CURVE('',#3727,#3727,#1506,.T.);
#4797=EDGE_CURVE('',#3726,#3728,#2444,.T.);
#4798=EDGE_CURVE('',#3728,#3728,#1507,.T.);
#4799=EDGE_CURVE('',#3711,#3727,#2445,.T.);
#6453=ORIENTED_EDGE('',*,*,#4650,.T.);
#6454=ORIENTED_EDGE('',*,*,#4651,.T.);
#6455=ORIENTED_EDGE('',*,*,#4652,.T.);
#6456=ORIENTED_EDGE('',*,*,#4653,.T.);
#6457=ORIENTED_EDGE('',*,*,#4654,.T.);
#6458=ORIENTED_EDGE('',*,*,#4655,.T.);
#6459=ORIENTED_EDGE('',*,*,#4654,.F.);
#6460=ORIENTED_EDGE('',*,*,#4656,.T.);
#6461=ORIENTED_EDGE('',*,*,#4657,.T.);
#6462=ORIENTED_EDGE('',*,*,#4658,.T.);
#6463=ORIENTED_EDGE('',*,*,#4650,.F.);
#6464=ORIENTED_EDGE('',*,*,#4659,.T.);
#6465=ORIENTED_EDGE('',*,*,#4660,.T.);
#6466=ORIENTED_EDGE('',*,*,#4661,.T.);
#6467=ORIENTED_EDGE('',*,*,#4657,.F.);
#6468=ORIENTED_EDGE('',*,*,#4662,.T.);
#6469=ORIENTED_EDGE('',*,*,#4663,.T.);
#6470=ORIENTED_EDGE('',*,*,#4664,.T.);
#6471=ORIENTED_EDGE('',*,*,#4660,.F.);
#6472=ORIENTED_EDGE('',*,*,#4665,.T.);
#6473=ORIENTED_EDGE('',*,*,#4666,.T.);
#6474=ORIENTED_EDGE('',*,*,#4667,.T.);
#6475=ORIENTED_EDGE('',*,*,#4663,.F.);
#6476=ORIENTED_EDGE('',*,*,#4668,.T.);
#6477=ORIENTED_EDGE('',*,*,#4669,.T.);
#6478=ORIENTED_EDGE('',*,*,#4670,.T.);
#6479=ORIENTED_EDGE('',*,*,#4666,.F.);
#6480=ORIENTED_EDGE('',*,*,#4671,.T.);
#6481=ORIENTED_EDGE('',*,*,#4672,.T.);
#6482=ORIENTED_EDGE('',*,*,#4673,.T.);
#6483=ORIENTED_EDGE('',*,*,#4669,.F.);
#6484=ORIENTED_EDGE('',*,*,#4674,.T.);
#6485=ORIENTED_EDGE('',*,*,#4675,.T.);
#6486=ORIENTED_EDGE('',*,*,#4676,.T.);
#6487=ORIENTED_EDGE('',*,*,#4672,.F.);
#6488=ORIENTED_EDGE('',*,*,#4677,.T.);
#6489=ORIENTED_EDGE('',*,*,#4678,.T.);
#6490=ORIENTED_EDGE('',*,*,#4679,.T.);
#6491=ORIENTED_EDGE('',*,*,#4675,.F.);
#6492=ORIENTED_EDGE('',*,*,#4680,.T.);
#6493=ORIENTED_EDGE('',*,*,#4681,.T.);
#6494=ORIENTED_EDGE('',*,*,#4682,.T.);
#6495=ORIENTED_EDGE('',*,*,#4678,.F.);
#6496=ORIENTED_EDGE('',*,*,#4683,.T.);
#6497=ORIENTED_EDGE('',*,*,#4684,.T.);
#6498=ORIENTED_EDGE('',*,*,#4685,.T.);
#6499=ORIENTED_EDGE('',*,*,#4681,.F.);
#6500=ORIENTED_EDGE('',*,*,#4686,.T.);
#6501=ORIENTED_EDGE('',*,*,#4687,.T.);
#6502=ORIENTED_EDGE('',*,*,#4688,.T.);
#6503=ORIENTED_EDGE('',*,*,#4684,.F.);
#6504=ORIENTED_EDGE('',*,*,#4689,.T.);
#6505=ORIENTED_EDGE('',*,*,#4690,.T.);
#6506=ORIENTED_EDGE('',*,*,#4691,.T.);
#6507=ORIENTED_EDGE('',*,*,#4687,.F.);
#6508=ORIENTED_EDGE('',*,*,#4692,.T.);
#6509=ORIENTED_EDGE('',*,*,#4693,.T.);
#6510=ORIENTED_EDGE('',*,*,#4694,.T.);
#6511=ORIENTED_EDGE('',*,*,#4690,.F.);
#6512=ORIENTED_EDGE('',*,*,#4695,.T.);
#6513=ORIENTED_EDGE('',*,*,#4696,.F.);
#6514=ORIENTED_EDGE('',*,*,#4697,.T.);
#6515=ORIENTED_EDGE('',*,*,#4698,.F.);
#6516=ORIENTED_EDGE('',*,*,#4699,.T.);
#6517=ORIENTED_EDGE('',*,*,#4700,.T.);
#6518=ORIENTED_EDGE('',*,*,#4701,.T.);
#6519=ORIENTED_EDGE('',*,*,#4702,.F.);
#6520=ORIENTED_EDGE('',*,*,#4703,.F.);
#6521=ORIENTED_EDGE('',*,*,#4704,.T.);
#6522=ORIENTED_EDGE('',*,*,#4705,.T.);
#6523=ORIENTED_EDGE('',*,*,#4700,.F.);
#6524=ORIENTED_EDGE('',*,*,#4706,.F.);
#6525=ORIENTED_EDGE('',*,*,#4707,.T.);
#6526=ORIENTED_EDGE('',*,*,#4708,.T.);
#6527=ORIENTED_EDGE('',*,*,#4704,.F.);
#6528=ORIENTED_EDGE('',*,*,#4709,.F.);
#6529=ORIENTED_EDGE('',*,*,#4710,.T.);
#6530=ORIENTED_EDGE('',*,*,#4711,.T.);
#6531=ORIENTED_EDGE('',*,*,#4707,.F.);
#6532=ORIENTED_EDGE('',*,*,#4712,.F.);
#6533=ORIENTED_EDGE('',*,*,#4713,.T.);
#6534=ORIENTED_EDGE('',*,*,#4714,.T.);
#6535=ORIENTED_EDGE('',*,*,#4710,.F.);
#6536=ORIENTED_EDGE('',*,*,#4715,.F.);
#6537=ORIENTED_EDGE('',*,*,#4716,.T.);
#6538=ORIENTED_EDGE('',*,*,#4717,.T.);
#6539=ORIENTED_EDGE('',*,*,#4713,.F.);
#6540=ORIENTED_EDGE('',*,*,#4718,.F.);
#6541=ORIENTED_EDGE('',*,*,#4719,.T.);
#6542=ORIENTED_EDGE('',*,*,#4720,.T.);
#6543=ORIENTED_EDGE('',*,*,#4716,.F.);
#6544=ORIENTED_EDGE('',*,*,#4721,.F.);
#6545=ORIENTED_EDGE('',*,*,#4722,.T.);
#6546=ORIENTED_EDGE('',*,*,#4723,.T.);
#6547=ORIENTED_EDGE('',*,*,#4719,.F.);
#6548=ORIENTED_EDGE('',*,*,#4724,.F.);
#6549=ORIENTED_EDGE('',*,*,#4725,.T.);
#6550=ORIENTED_EDGE('',*,*,#4726,.T.);
#6551=ORIENTED_EDGE('',*,*,#4722,.F.);
#6552=ORIENTED_EDGE('',*,*,#4727,.F.);
#6553=ORIENTED_EDGE('',*,*,#4728,.T.);
#6554=ORIENTED_EDGE('',*,*,#4729,.T.);
#6555=ORIENTED_EDGE('',*,*,#4725,.F.);
#6556=ORIENTED_EDGE('',*,*,#4730,.F.);
#6557=ORIENTED_EDGE('',*,*,#4731,.T.);
#6558=ORIENTED_EDGE('',*,*,#4732,.T.);
#6559=ORIENTED_EDGE('',*,*,#4728,.F.);
#6560=ORIENTED_EDGE('',*,*,#4733,.F.);
#6561=ORIENTED_EDGE('',*,*,#4734,.T.);
#6562=ORIENTED_EDGE('',*,*,#4735,.T.);
#6563=ORIENTED_EDGE('',*,*,#4731,.F.);
#6564=ORIENTED_EDGE('',*,*,#4736,.F.);
#6565=ORIENTED_EDGE('',*,*,#4737,.T.);
#6566=ORIENTED_EDGE('',*,*,#4738,.T.);
#6567=ORIENTED_EDGE('',*,*,#4734,.F.);
#6568=ORIENTED_EDGE('',*,*,#4739,.F.);
#6569=ORIENTED_EDGE('',*,*,#4740,.T.);
#6570=ORIENTED_EDGE('',*,*,#4741,.T.);
#6571=ORIENTED_EDGE('',*,*,#4737,.F.);
#6572=ORIENTED_EDGE('',*,*,#4742,.F.);
#6573=ORIENTED_EDGE('',*,*,#4743,.T.);
#6574=ORIENTED_EDGE('',*,*,#4744,.T.);
#6575=ORIENTED_EDGE('',*,*,#4740,.F.);
#6576=ORIENTED_EDGE('',*,*,#4745,.F.);
#6577=ORIENTED_EDGE('',*,*,#4746,.F.);
#6578=ORIENTED_EDGE('',*,*,#4747,.F.);
#6579=ORIENTED_EDGE('',*,*,#4748,.F.);
#6580=ORIENTED_EDGE('',*,*,#4749,.T.);
#6581=ORIENTED_EDGE('',*,*,#4652,.F.);
#6582=ORIENTED_EDGE('',*,*,#4750,.T.);
#6583=ORIENTED_EDGE('',*,*,#4702,.T.);
#6584=ORIENTED_EDGE('',*,*,#4751,.T.);
#6585=ORIENTED_EDGE('',*,*,#4746,.T.);
#6586=ORIENTED_EDGE('',*,*,#4752,.T.);
#6587=ORIENTED_EDGE('',*,*,#4743,.F.);
#6588=ORIENTED_EDGE('',*,*,#4753,.F.);
#6589=ORIENTED_EDGE('',*,*,#4751,.F.);
#6590=ORIENTED_EDGE('',*,*,#4701,.F.);
#6591=ORIENTED_EDGE('',*,*,#4705,.F.);
#6592=ORIENTED_EDGE('',*,*,#4708,.F.);
#6593=ORIENTED_EDGE('',*,*,#4711,.F.);
#6594=ORIENTED_EDGE('',*,*,#4714,.F.);
#6595=ORIENTED_EDGE('',*,*,#4717,.F.);
#6596=ORIENTED_EDGE('',*,*,#4720,.F.);
#6597=ORIENTED_EDGE('',*,*,#4723,.F.);
#6598=ORIENTED_EDGE('',*,*,#4726,.F.);
#6599=ORIENTED_EDGE('',*,*,#4729,.F.);
#6600=ORIENTED_EDGE('',*,*,#4732,.F.);
#6601=ORIENTED_EDGE('',*,*,#4735,.F.);
#6602=ORIENTED_EDGE('',*,*,#4738,.F.);
#6603=ORIENTED_EDGE('',*,*,#4741,.F.);
#6604=ORIENTED_EDGE('',*,*,#4744,.F.);
#6605=ORIENTED_EDGE('',*,*,#4752,.F.);
#6606=ORIENTED_EDGE('',*,*,#4749,.F.);
#6607=ORIENTED_EDGE('',*,*,#4754,.F.);
#6608=ORIENTED_EDGE('',*,*,#4697,.F.);
#6609=ORIENTED_EDGE('',*,*,#4755,.F.);
#6610=ORIENTED_EDGE('',*,*,#4695,.F.);
#6611=ORIENTED_EDGE('',*,*,#4692,.F.);
#6612=ORIENTED_EDGE('',*,*,#4689,.F.);
#6613=ORIENTED_EDGE('',*,*,#4686,.F.);
#6614=ORIENTED_EDGE('',*,*,#4683,.F.);
#6615=ORIENTED_EDGE('',*,*,#4680,.F.);
#6616=ORIENTED_EDGE('',*,*,#4677,.F.);
#6617=ORIENTED_EDGE('',*,*,#4674,.F.);
#6618=ORIENTED_EDGE('',*,*,#4671,.F.);
#6619=ORIENTED_EDGE('',*,*,#4668,.F.);
#6620=ORIENTED_EDGE('',*,*,#4665,.F.);
#6621=ORIENTED_EDGE('',*,*,#4662,.F.);
#6622=ORIENTED_EDGE('',*,*,#4659,.F.);
#6623=ORIENTED_EDGE('',*,*,#4656,.F.);
#6624=ORIENTED_EDGE('',*,*,#4653,.F.);
#6625=ORIENTED_EDGE('',*,*,#4750,.F.);
#6626=ORIENTED_EDGE('',*,*,#4651,.F.);
#6627=ORIENTED_EDGE('',*,*,#4658,.F.);
#6628=ORIENTED_EDGE('',*,*,#4661,.F.);
#6629=ORIENTED_EDGE('',*,*,#4664,.F.);
#6630=ORIENTED_EDGE('',*,*,#4667,.F.);
#6631=ORIENTED_EDGE('',*,*,#4670,.F.);
#6632=ORIENTED_EDGE('',*,*,#4673,.F.);
#6633=ORIENTED_EDGE('',*,*,#4676,.F.);
#6634=ORIENTED_EDGE('',*,*,#4679,.F.);
#6635=ORIENTED_EDGE('',*,*,#4682,.F.);
#6636=ORIENTED_EDGE('',*,*,#4685,.F.);
#6637=ORIENTED_EDGE('',*,*,#4688,.F.);
#6638=ORIENTED_EDGE('',*,*,#4691,.F.);
#6639=ORIENTED_EDGE('',*,*,#4694,.F.);
#6640=ORIENTED_EDGE('',*,*,#4756,.F.);
#6641=ORIENTED_EDGE('',*,*,#4699,.F.);
#6642=ORIENTED_EDGE('',*,*,#4757,.F.);
#6643=ORIENTED_EDGE('',*,*,#4747,.T.);
#6644=ORIENTED_EDGE('',*,*,#4753,.T.);
#6645=ORIENTED_EDGE('',*,*,#4745,.T.);
#6646=ORIENTED_EDGE('',*,*,#4742,.T.);
#6647=ORIENTED_EDGE('',*,*,#4739,.T.);
#6648=ORIENTED_EDGE('',*,*,#4736,.T.);
#6649=ORIENTED_EDGE('',*,*,#4733,.T.);
#6650=ORIENTED_EDGE('',*,*,#4730,.T.);
#6651=ORIENTED_EDGE('',*,*,#4727,.T.);
#6652=ORIENTED_EDGE('',*,*,#4724,.T.);
#6653=ORIENTED_EDGE('',*,*,#4721,.T.);
#6654=ORIENTED_EDGE('',*,*,#4718,.T.);
#6655=ORIENTED_EDGE('',*,*,#4715,.T.);
#6656=ORIENTED_EDGE('',*,*,#4712,.T.);
#6657=ORIENTED_EDGE('',*,*,#4709,.T.);
#6658=ORIENTED_EDGE('',*,*,#4706,.T.);
#6659=ORIENTED_EDGE('',*,*,#4703,.T.);
#6660=ORIENTED_EDGE('',*,*,#4696,.T.);
#6661=ORIENTED_EDGE('',*,*,#4756,.T.);
#6662=ORIENTED_EDGE('',*,*,#4693,.F.);
#6663=ORIENTED_EDGE('',*,*,#4755,.T.);
#6664=ORIENTED_EDGE('',*,*,#4655,.F.);
#6665=ORIENTED_EDGE('',*,*,#4758,.T.);
#6666=ORIENTED_EDGE('',*,*,#4759,.T.);
#6667=ORIENTED_EDGE('',*,*,#4760,.F.);
#6668=ORIENTED_EDGE('',*,*,#4761,.F.);
#6669=ORIENTED_EDGE('',*,*,#4762,.T.);
#6670=ORIENTED_EDGE('',*,*,#4763,.T.);
#6671=ORIENTED_EDGE('',*,*,#4764,.F.);
#6672=ORIENTED_EDGE('',*,*,#4759,.F.);
#6673=ORIENTED_EDGE('',*,*,#4765,.T.);
#6674=ORIENTED_EDGE('',*,*,#4766,.T.);
#6675=ORIENTED_EDGE('',*,*,#4767,.F.);
#6676=ORIENTED_EDGE('',*,*,#4763,.F.);
#6677=ORIENTED_EDGE('',*,*,#4768,.T.);
#6678=ORIENTED_EDGE('',*,*,#4761,.T.);
#6679=ORIENTED_EDGE('',*,*,#4769,.F.);
#6680=ORIENTED_EDGE('',*,*,#4766,.F.);
#6681=ORIENTED_EDGE('',*,*,#4768,.F.);
#6682=ORIENTED_EDGE('',*,*,#4765,.F.);
#6683=ORIENTED_EDGE('',*,*,#4762,.F.);
#6684=ORIENTED_EDGE('',*,*,#4758,.F.);
#6685=ORIENTED_EDGE('',*,*,#4770,.T.);
#6686=ORIENTED_EDGE('',*,*,#4771,.T.);
#6687=ORIENTED_EDGE('',*,*,#4772,.F.);
#6688=ORIENTED_EDGE('',*,*,#4771,.F.);
#6689=ORIENTED_EDGE('',*,*,#4773,.F.);
#6690=ORIENTED_EDGE('',*,*,#4770,.F.);
#6691=ORIENTED_EDGE('',*,*,#4774,.F.);
#6692=ORIENTED_EDGE('',*,*,#4772,.T.);
#6693=ORIENTED_EDGE('',*,*,#4775,.F.);
#6694=ORIENTED_EDGE('',*,*,#4776,.T.);
#6695=ORIENTED_EDGE('',*,*,#4774,.T.);
#6696=ORIENTED_EDGE('',*,*,#4776,.F.);
#6697=ORIENTED_EDGE('',*,*,#4777,.F.);
#6698=ORIENTED_EDGE('',*,*,#4778,.T.);
#6699=ORIENTED_EDGE('',*,*,#4779,.F.);
#6700=ORIENTED_EDGE('',*,*,#4780,.F.);
#6701=ORIENTED_EDGE('',*,*,#4781,.F.);
#6702=ORIENTED_EDGE('',*,*,#4780,.T.);
#6703=ORIENTED_EDGE('',*,*,#4782,.F.);
#6704=ORIENTED_EDGE('',*,*,#4783,.F.);
#6705=ORIENTED_EDGE('',*,*,#4784,.F.);
#6706=ORIENTED_EDGE('',*,*,#4783,.T.);
#6707=ORIENTED_EDGE('',*,*,#4785,.F.);
#6708=ORIENTED_EDGE('',*,*,#4786,.F.);
#6709=ORIENTED_EDGE('',*,*,#4787,.F.);
#6710=ORIENTED_EDGE('',*,*,#4786,.T.);
#6711=ORIENTED_EDGE('',*,*,#4788,.F.);
#6712=ORIENTED_EDGE('',*,*,#4789,.F.);
#6713=ORIENTED_EDGE('',*,*,#4790,.F.);
#6714=ORIENTED_EDGE('',*,*,#4789,.T.);
#6715=ORIENTED_EDGE('',*,*,#4791,.F.);
#6716=ORIENTED_EDGE('',*,*,#4792,.F.);
#6717=ORIENTED_EDGE('',*,*,#4793,.F.);
#6718=ORIENTED_EDGE('',*,*,#4792,.T.);
#6719=ORIENTED_EDGE('',*,*,#4794,.F.);
#6720=ORIENTED_EDGE('',*,*,#4778,.F.);
#6721=ORIENTED_EDGE('',*,*,#4794,.T.);
#6722=ORIENTED_EDGE('',*,*,#4791,.T.);
#6723=ORIENTED_EDGE('',*,*,#4788,.T.);
#6724=ORIENTED_EDGE('',*,*,#4785,.T.);
#6725=ORIENTED_EDGE('',*,*,#4782,.T.);
#6726=ORIENTED_EDGE('',*,*,#4779,.T.);
#6727=ORIENTED_EDGE('',*,*,#4757,.T.);
#6728=ORIENTED_EDGE('',*,*,#4698,.T.);
#6729=ORIENTED_EDGE('',*,*,#4754,.T.);
#6730=ORIENTED_EDGE('',*,*,#4748,.T.);
#6731=ORIENTED_EDGE('',*,*,#4795,.T.);
#6732=ORIENTED_EDGE('',*,*,#4796,.F.);
#6733=ORIENTED_EDGE('',*,*,#4795,.F.);
#6734=ORIENTED_EDGE('',*,*,#4797,.T.);
#6735=ORIENTED_EDGE('',*,*,#4798,.T.);
#6736=ORIENTED_EDGE('',*,*,#4797,.F.);
#6737=ORIENTED_EDGE('',*,*,#4798,.F.);
#6738=ORIENTED_EDGE('',*,*,#4760,.T.);
#6739=ORIENTED_EDGE('',*,*,#4764,.T.);
#6740=ORIENTED_EDGE('',*,*,#4767,.T.);
#6741=ORIENTED_EDGE('',*,*,#4769,.T.);
#6742=ORIENTED_EDGE('',*,*,#4773,.T.);
#6743=ORIENTED_EDGE('',*,*,#4799,.T.);
#6744=ORIENTED_EDGE('',*,*,#4796,.T.);
#6745=ORIENTED_EDGE('',*,*,#4799,.F.);
#6746=ORIENTED_EDGE('',*,*,#4775,.T.);
#6747=ORIENTED_EDGE('',*,*,#4777,.T.);
#6748=ORIENTED_EDGE('',*,*,#4781,.T.);
#6749=ORIENTED_EDGE('',*,*,#4784,.T.);
#6750=ORIENTED_EDGE('',*,*,#4787,.T.);
#6751=ORIENTED_EDGE('',*,*,#4790,.T.);
#6752=ORIENTED_EDGE('',*,*,#4793,.T.);
#8036=CYLINDRICAL_SURFACE('',#9114,1.666);
#8037=CYLINDRICAL_SURFACE('',#9117,1.666);
#8038=CYLINDRICAL_SURFACE('',#9118,1.666);
#8039=CYLINDRICAL_SURFACE('',#9119,1.666);
#8040=CYLINDRICAL_SURFACE('',#9120,1.666);
#8041=CYLINDRICAL_SURFACE('',#9121,1.666);
#8042=CYLINDRICAL_SURFACE('',#9122,1.666);
#8043=CYLINDRICAL_SURFACE('',#9123,1.666);
#8044=CYLINDRICAL_SURFACE('',#9124,1.666);
#8045=CYLINDRICAL_SURFACE('',#9125,1.666);
#8046=CYLINDRICAL_SURFACE('',#9126,1.666);
#8047=CYLINDRICAL_SURFACE('',#9127,1.666);
#8048=CYLINDRICAL_SURFACE('',#9128,1.666);
#8049=CYLINDRICAL_SURFACE('',#9129,1.666);
#8050=CYLINDRICAL_SURFACE('',#9130,1.666);
#8051=CYLINDRICAL_SURFACE('',#9132,2.05475);
#8052=CYLINDRICAL_SURFACE('',#9134,2.05475);
#8053=CYLINDRICAL_SURFACE('',#9135,2.05475);
#8054=CYLINDRICAL_SURFACE('',#9136,2.05475);
#8055=CYLINDRICAL_SURFACE('',#9137,2.05475);
#8056=CYLINDRICAL_SURFACE('',#9138,2.05475);
#8057=CYLINDRICAL_SURFACE('',#9139,2.05475);
#8058=CYLINDRICAL_SURFACE('',#9140,2.05475);
#8059=CYLINDRICAL_SURFACE('',#9141,2.05475);
#8060=CYLINDRICAL_SURFACE('',#9142,2.05475);
#8061=CYLINDRICAL_SURFACE('',#9143,2.05475);
#8062=CYLINDRICAL_SURFACE('',#9144,2.05475);
#8063=CYLINDRICAL_SURFACE('',#9145,2.05475);
#8064=CYLINDRICAL_SURFACE('',#9146,2.05475);
#8065=CYLINDRICAL_SURFACE('',#9147,2.05475);
#8066=CYLINDRICAL_SURFACE('',#9148,2.05475);
#8067=CYLINDRICAL_SURFACE('',#9151,2.05475);
#8068=CYLINDRICAL_SURFACE('',#9152,1.666);
#8069=CYLINDRICAL_SURFACE('',#9159,3.);
#8070=CYLINDRICAL_SURFACE('',#9166,4.);
#8071=CYLINDRICAL_SURFACE('',#9178,10.);
#8072=CYLINDRICAL_SURFACE('',#9181,4.);
#8391=ADVANCED_FACE('',(#643),#8036,.F.);
#8392=ADVANCED_FACE('',(#644),#8037,.F.);
#8393=ADVANCED_FACE('',(#645),#8038,.F.);
#8394=ADVANCED_FACE('',(#646),#8039,.F.);
#8395=ADVANCED_FACE('',(#647),#8040,.F.);
#8396=ADVANCED_FACE('',(#648),#8041,.F.);
#8397=ADVANCED_FACE('',(#649),#8042,.F.);
#8398=ADVANCED_FACE('',(#650),#8043,.F.);
#8399=ADVANCED_FACE('',(#651),#8044,.F.);
#8400=ADVANCED_FACE('',(#652),#8045,.F.);
#8401=ADVANCED_FACE('',(#653),#8046,.F.);
#8402=ADVANCED_FACE('',(#654),#8047,.F.);
#8403=ADVANCED_FACE('',(#655),#8048,.F.);
#8404=ADVANCED_FACE('',(#656),#8049,.F.);
#8405=ADVANCED_FACE('',(#657),#8050,.F.);
#8406=ADVANCED_FACE('',(#658),#8051,.F.);
#8407=ADVANCED_FACE('',(#659),#8052,.F.);
#8408=ADVANCED_FACE('',(#660),#8053,.F.);
#8409=ADVANCED_FACE('',(#661),#8054,.F.);
#8410=ADVANCED_FACE('',(#662),#8055,.F.);
#8411=ADVANCED_FACE('',(#663),#8056,.F.);
#8412=ADVANCED_FACE('',(#664),#8057,.F.);
#8413=ADVANCED_FACE('',(#665),#8058,.F.);
#8414=ADVANCED_FACE('',(#666),#8059,.F.);
#8415=ADVANCED_FACE('',(#667),#8060,.F.);
#8416=ADVANCED_FACE('',(#668),#8061,.F.);
#8417=ADVANCED_FACE('',(#669),#8062,.F.);
#8418=ADVANCED_FACE('',(#670),#8063,.F.);
#8419=ADVANCED_FACE('',(#671),#8064,.F.);
#8420=ADVANCED_FACE('',(#672),#8065,.F.);
#8421=ADVANCED_FACE('',(#673),#8066,.F.);
#8422=ADVANCED_FACE('',(#674),#345,.T.);
#8423=ADVANCED_FACE('',(#675),#8067,.F.);
#8424=ADVANCED_FACE('',(#676),#301,.F.);
#8425=ADVANCED_FACE('',(#677),#302,.F.);
#8426=ADVANCED_FACE('',(#678),#8068,.F.);
#8427=ADVANCED_FACE('',(#679),#346,.F.);
#8428=ADVANCED_FACE('',(#680),#347,.F.);
#8429=ADVANCED_FACE('',(#681),#348,.F.);
#8430=ADVANCED_FACE('',(#682),#349,.F.);
#8431=ADVANCED_FACE('',(#683),#350,.F.);
#8432=ADVANCED_FACE('',(#684),#351,.F.);
#8433=ADVANCED_FACE('',(#685),#8069,.T.);
#8434=ADVANCED_FACE('',(#686,#252),#352,.F.);
#8435=ADVANCED_FACE('',(#687,#253),#353,.F.);
#8436=ADVANCED_FACE('',(#688),#8070,.T.);
#8437=ADVANCED_FACE('',(#689),#354,.T.);
#8438=ADVANCED_FACE('',(#690),#355,.T.);
#8439=ADVANCED_FACE('',(#691),#356,.T.);
#8440=ADVANCED_FACE('',(#692),#357,.T.);
#8441=ADVANCED_FACE('',(#693),#358,.T.);
#8442=ADVANCED_FACE('',(#694),#359,.T.);
#8443=ADVANCED_FACE('',(#695,#254),#360,.T.);
#8444=ADVANCED_FACE('',(#696,#255),#361,.T.);
#8445=ADVANCED_FACE('',(#697),#8071,.T.);
#8446=ADVANCED_FACE('',(#698,#256),#362,.F.);
#8447=ADVANCED_FACE('',(#699),#8072,.T.);
#8448=ADVANCED_FACE('',(#700,#257),#363,.T.);
#8678=CLOSED_SHELL('',(#8391,#8392,#8393,#8394,#8395,#8396,#8397,#8398,
#8399,#8400,#8401,#8402,#8403,#8404,#8405,#8406,#8407,#8408,#8409,#8410,
#8411,#8412,#8413,#8414,#8415,#8416,#8417,#8418,#8419,#8420,#8421,#8422,
#8423,#8424,#8425,#8426,#8427,#8428,#8429,#8430,#8431,#8432,#8433,#8434,
#8435,#8436,#8437,#8438,#8439,#8440,#8441,#8442,#8443,#8444,#8445,#8446,
#8447,#8448));
#9113=AXIS2_PLACEMENT_3D('',#21745,#10176,#10177);
#9114=AXIS2_PLACEMENT_3D('',#21746,#10178,#10179);
#9115=AXIS2_PLACEMENT_3D('',#21771,#10181,#10182);
#9116=AXIS2_PLACEMENT_3D('',#21779,#10184,#10185);
#9117=AXIS2_PLACEMENT_3D('',#21802,#10186,#10187);
#9118=AXIS2_PLACEMENT_3D('',#21853,#10189,#10190);
#9119=AXIS2_PLACEMENT_3D('',#21901,#10192,#10193);
#9120=AXIS2_PLACEMENT_3D('',#21952,#10195,#10196);
#9121=AXIS2_PLACEMENT_3D('',#22003,#10198,#10199);
#9122=AXIS2_PLACEMENT_3D('',#22051,#10201,#10202);
#9123=AXIS2_PLACEMENT_3D('',#22099,#10204,#10205);
#9124=AXIS2_PLACEMENT_3D('',#22150,#10207,#10208);
#9125=AXIS2_PLACEMENT_3D('',#22198,#10210,#10211);
#9126=AXIS2_PLACEMENT_3D('',#22246,#10213,#10214);
#9127=AXIS2_PLACEMENT_3D('',#22297,#10216,#10217);
#9128=AXIS2_PLACEMENT_3D('',#22348,#10219,#10220);
#9129=AXIS2_PLACEMENT_3D('',#22396,#10222,#10223);
#9130=AXIS2_PLACEMENT_3D('',#22447,#10225,#10226);
#9131=AXIS2_PLACEMENT_3D('',#22466,#10228,#10229);
#9132=AXIS2_PLACEMENT_3D('',#22486,#10230,#10231);
#9133=AXIS2_PLACEMENT_3D('',#22498,#10233,#10234);
#9134=AXIS2_PLACEMENT_3D('',#22506,#10235,#10236);
#9135=AXIS2_PLACEMENT_3D('',#22530,#10238,#10239);
#9136=AXIS2_PLACEMENT_3D('',#22555,#10241,#10242);
#9137=AXIS2_PLACEMENT_3D('',#22580,#10244,#10245);
#9138=AXIS2_PLACEMENT_3D('',#22604,#10247,#10248);
#9139=AXIS2_PLACEMENT_3D('',#22629,#10250,#10251);
#9140=AXIS2_PLACEMENT_3D('',#22653,#10253,#10254);
#9141=AXIS2_PLACEMENT_3D('',#22678,#10256,#10257);
#9142=AXIS2_PLACEMENT_3D('',#22703,#10259,#10260);
#9143=AXIS2_PLACEMENT_3D('',#22727,#10262,#10263);
#9144=AXIS2_PLACEMENT_3D('',#22752,#10265,#10266);
#9145=AXIS2_PLACEMENT_3D('',#22776,#10268,#10269);
#9146=AXIS2_PLACEMENT_3D('',#22801,#10271,#10272);
#9147=AXIS2_PLACEMENT_3D('',#22826,#10274,#10275);
#9148=AXIS2_PLACEMENT_3D('',#22850,#10277,#10278);
#9149=AXIS2_PLACEMENT_3D('',#22861,#10280,#10281);
#9150=AXIS2_PLACEMENT_3D('',#22867,#10282,#10283);
#9151=AXIS2_PLACEMENT_3D('',#23041,#10284,#10285);
#9152=AXIS2_PLACEMENT_3D('',#24109,#10286,#10287);
#9153=AXIS2_PLACEMENT_3D('',#24110,#10288,#10289);
#9154=AXIS2_PLACEMENT_3D('',#24111,#10290,#10291);
#9155=AXIS2_PLACEMENT_3D('',#24120,#10296,#10297);
#9156=AXIS2_PLACEMENT_3D('',#24126,#10301,#10302);
#9157=AXIS2_PLACEMENT_3D('',#24132,#10306,#10307);
#9158=AXIS2_PLACEMENT_3D('',#24135,#10310,#10311);
#9159=AXIS2_PLACEMENT_3D('',#24136,#10312,#10313);
#9160=AXIS2_PLACEMENT_3D('',#24138,#10314,#10315);
#9161=AXIS2_PLACEMENT_3D('',#24141,#10317,#10318);
#9162=AXIS2_PLACEMENT_3D('',#24142,#10319,#10320);
#9163=AXIS2_PLACEMENT_3D('',#24144,#10321,#10322);
#9164=AXIS2_PLACEMENT_3D('',#24145,#10323,#10324);
#9165=AXIS2_PLACEMENT_3D('',#24147,#10325,#10326);
#9166=AXIS2_PLACEMENT_3D('',#24148,#10327,#10328);
#9167=AXIS2_PLACEMENT_3D('',#24150,#10329,#10330);
#9168=AXIS2_PLACEMENT_3D('',#24152,#10332,#10333);
#9169=AXIS2_PLACEMENT_3D('',#24161,#10338,#10339);
#9170=AXIS2_PLACEMENT_3D('',#24167,#10343,#10344);
#9171=AXIS2_PLACEMENT_3D('',#24173,#10348,#10349);
#9172=AXIS2_PLACEMENT_3D('',#24179,#10353,#10354);
#9173=AXIS2_PLACEMENT_3D('',#24185,#10358,#10359);
#9174=AXIS2_PLACEMENT_3D('',#24188,#10362,#10363);
#9175=AXIS2_PLACEMENT_3D('',#24189,#10364,#10365);
#9176=AXIS2_PLACEMENT_3D('',#24191,#10366,#10367);
#9177=AXIS2_PLACEMENT_3D('',#24193,#10368,#10369);
#9178=AXIS2_PLACEMENT_3D('',#24194,#10370,#10371);
#9179=AXIS2_PLACEMENT_3D('',#24197,#10373,#10374);
#9180=AXIS2_PLACEMENT_3D('',#24198,#10375,#10376);
#9181=AXIS2_PLACEMENT_3D('',#24199,#10377,#10378);
#9182=AXIS2_PLACEMENT_3D('',#24201,#10380,#10381);
#10176=DIRECTION('axis',(0.,0.,1.));
#10177=DIRECTION('refdir',(1.,0.,0.));
#10178=DIRECTION('center_axis',(0.,0.,-1.));
#10179=DIRECTION('ref_axis',(1.,0.,0.));
#10180=DIRECTION('',(0.,0.,-1.));
#10181=DIRECTION('center_axis',(0.,0.,1.));
#10182=DIRECTION('ref_axis',(1.,0.,0.));
#10183=DIRECTION('',(0.,0.,-1.));
#10184=DIRECTION('center_axis',(0.,0.,1.));
#10185=DIRECTION('ref_axis',(1.,0.,0.));
#10186=DIRECTION('center_axis',(0.,0.,-1.));
#10187=DIRECTION('ref_axis',(1.,0.,0.));
#10188=DIRECTION('',(0.,0.,-1.));
#10189=DIRECTION('center_axis',(0.,0.,-1.));
#10190=DIRECTION('ref_axis',(1.,0.,0.));
#10191=DIRECTION('',(0.,0.,-1.));
#10192=DIRECTION('center_axis',(0.,0.,-1.));
#10193=DIRECTION('ref_axis',(1.,0.,0.));
#10194=DIRECTION('',(0.,0.,-1.));
#10195=DIRECTION('center_axis',(0.,0.,-1.));
#10196=DIRECTION('ref_axis',(1.,0.,0.));
#10197=DIRECTION('',(0.,0.,-1.));
#10198=DIRECTION('center_axis',(0.,0.,-1.));
#10199=DIRECTION('ref_axis',(1.,0.,0.));
#10200=DIRECTION('',(0.,0.,-1.));
#10201=DIRECTION('center_axis',(0.,0.,-1.));
#10202=DIRECTION('ref_axis',(1.,0.,0.));
#10203=DIRECTION('',(0.,0.,-1.));
#10204=DIRECTION('center_axis',(0.,0.,-1.));
#10205=DIRECTION('ref_axis',(1.,0.,0.));
#10206=DIRECTION('',(0.,0.,-1.));
#10207=DIRECTION('center_axis',(0.,0.,-1.));
#10208=DIRECTION('ref_axis',(1.,0.,0.));
#10209=DIRECTION('',(0.,0.,-1.));
#10210=DIRECTION('center_axis',(0.,0.,-1.));
#10211=DIRECTION('ref_axis',(1.,0.,0.));
#10212=DIRECTION('',(0.,0.,-1.));
#10213=DIRECTION('center_axis',(0.,0.,-1.));
#10214=DIRECTION('ref_axis',(1.,0.,0.));
#10215=DIRECTION('',(0.,0.,-1.));
#10216=DIRECTION('center_axis',(0.,0.,-1.));
#10217=DIRECTION('ref_axis',(1.,0.,0.));
#10218=DIRECTION('',(0.,0.,-1.));
#10219=DIRECTION('center_axis',(0.,0.,-1.));
#10220=DIRECTION('ref_axis',(1.,0.,0.));
#10221=DIRECTION('',(0.,0.,-1.));
#10222=DIRECTION('center_axis',(0.,0.,-1.));
#10223=DIRECTION('ref_axis',(1.,0.,0.));
#10224=DIRECTION('',(0.,0.,-1.));
#10225=DIRECTION('center_axis',(0.,0.,-1.));
#10226=DIRECTION('ref_axis',(0.938434895654951,-0.34545614282725,0.));
#10227=DIRECTION('',(0.,0.,-1.));
#10228=DIRECTION('center_axis',(0.,0.,-1.));
#10229=DIRECTION('ref_axis',(1.,0.,0.));
#10230=DIRECTION('center_axis',(0.,0.,-1.));
#10231=DIRECTION('ref_axis',(0.0179472551277058,0.999838935045731,0.));
#10232=DIRECTION('',(1.22464679914735E-16,-9.43079471310298E-30,-1.));
#10233=DIRECTION('center_axis',(0.,0.,1.));
#10234=DIRECTION('ref_axis',(1.,-7.68858181953524E-14,0.));
#10235=DIRECTION('center_axis',(0.,0.,-1.));
#10236=DIRECTION('ref_axis',(1.,-7.68858181953524E-14,0.));
#10237=DIRECTION('',(1.22464679914735E-16,-9.43079471310298E-30,-1.));
#10238=DIRECTION('center_axis',(0.,0.,-1.));
#10239=DIRECTION('ref_axis',(1.,-7.68858181953524E-14,0.));
#10240=DIRECTION('',(1.22464679914735E-16,-9.43079471310298E-30,-1.));
#10241=DIRECTION('center_axis',(0.,0.,-1.));
#10242=DIRECTION('ref_axis',(1.,-7.68858181953524E-14,0.));
#10243=DIRECTION('',(1.22464679914735E-16,-9.43079471310298E-30,-1.));
#10244=DIRECTION('center_axis',(0.,0.,-1.));
#10245=DIRECTION('ref_axis',(1.,-7.68858181953524E-14,0.));
#10246=DIRECTION('',(1.22464679914735E-16,-9.43079471310298E-30,-1.));
#10247=DIRECTION('center_axis',(0.,0.,-1.));
#10248=DIRECTION('ref_axis',(1.,-7.68858181953524E-14,0.));
#10249=DIRECTION('',(1.22464679914735E-16,-9.43079471310298E-30,-1.));
#10250=DIRECTION('center_axis',(0.,0.,-1.));
#10251=DIRECTION('ref_axis',(1.,-7.68858181953524E-14,0.));
#10252=DIRECTION('',(1.22464679914735E-16,-9.43079471310298E-30,-1.));
#10253=DIRECTION('center_axis',(0.,0.,-1.));
#10254=DIRECTION('ref_axis',(1.,-7.68858181953524E-14,0.));
#10255=DIRECTION('',(1.22464679914735E-16,-9.43079471310298E-30,-1.));
#10256=DIRECTION('center_axis',(0.,0.,-1.));
#10257=DIRECTION('ref_axis',(1.,-7.68858181953524E-14,0.));
#10258=DIRECTION('',(1.22464679914735E-16,-9.43079471310298E-30,-1.));
#10259=DIRECTION('center_axis',(0.,0.,-1.));
#10260=DIRECTION('ref_axis',(1.,-7.68858181953524E-14,0.));
#10261=DIRECTION('',(1.22464679914735E-16,-9.43079471310298E-30,-1.));
#10262=DIRECTION('center_axis',(0.,0.,-1.));
#10263=DIRECTION('ref_axis',(1.,-7.68858181953524E-14,0.));
#10264=DIRECTION('',(1.22464679914735E-16,-9.43079471310298E-30,-1.));
#10265=DIRECTION('center_axis',(0.,0.,-1.));
#10266=DIRECTION('ref_axis',(1.,-7.68858181953524E-14,0.));
#10267=DIRECTION('',(1.22464679914735E-16,-9.43079471310298E-30,-1.));
#10268=DIRECTION('center_axis',(0.,0.,-1.));
#10269=DIRECTION('ref_axis',(1.,-7.68858181953524E-14,0.));
#10270=DIRECTION('',(1.22464679914735E-16,-9.43079471310298E-30,-1.));
#10271=DIRECTION('center_axis',(0.,0.,-1.));
#10272=DIRECTION('ref_axis',(1.,-7.68858181953524E-14,0.));
#10273=DIRECTION('',(1.22464679914735E-16,-9.43079471310298E-30,-1.));
#10274=DIRECTION('center_axis',(0.,0.,-1.));
#10275=DIRECTION('ref_axis',(1.,-7.68858181953524E-14,0.));
#10276=DIRECTION('',(1.22464679914735E-16,-9.43079471310298E-30,-1.));
#10277=DIRECTION('center_axis',(0.,0.,-1.));
#10278=DIRECTION('ref_axis',(-0.609350010373174,-0.792901358844978,0.));
#10279=DIRECTION('',(1.22464679914735E-16,-9.43079471310298E-30,-1.));
#10280=DIRECTION('center_axis',(0.,0.,-1.));
#10281=DIRECTION('ref_axis',(1.,-7.68858181953524E-14,0.));
#10282=DIRECTION('center_axis',(0.,0.,1.));
#10283=DIRECTION('ref_axis',(1.,0.,0.));
#10284=DIRECTION('center_axis',(0.,0.,-1.));
#10285=DIRECTION('ref_axis',(1.,-7.68858181953524E-14,0.));
#10286=DIRECTION('center_axis',(0.,0.,-1.));
#10287=DIRECTION('ref_axis',(1.,0.,0.));
#10288=DIRECTION('center_axis',(0.,0.,-1.));
#10289=DIRECTION('ref_axis',(1.,0.,0.));
#10290=DIRECTION('center_axis',(0.,-1.,0.));
#10291=DIRECTION('ref_axis',(-1.,0.,0.));
#10292=DIRECTION('',(1.,0.,0.));
#10293=DIRECTION('',(0.,0.,-1.));
#10294=DIRECTION('',(1.,0.,0.));
#10295=DIRECTION('',(0.,0.,-1.));
#10296=DIRECTION('center_axis',(1.,0.,0.));
#10297=DIRECTION('ref_axis',(0.,-1.,0.));
#10298=DIRECTION('',(0.,1.,0.));
#10299=DIRECTION('',(0.,0.,-1.));
#10300=DIRECTION('',(0.,1.,0.));
#10301=DIRECTION('center_axis',(0.,1.,0.));
#10302=DIRECTION('ref_axis',(1.,0.,0.));
#10303=DIRECTION('',(-1.,0.,0.));
#10304=DIRECTION('',(0.,0.,-1.));
#10305=DIRECTION('',(-1.,0.,0.));
#10306=DIRECTION('center_axis',(-1.,0.,0.));
#10307=DIRECTION('ref_axis',(0.,1.,0.));
#10308=DIRECTION('',(0.,-1.,0.));
#10309=DIRECTION('',(0.,-1.,0.));
#10310=DIRECTION('center_axis',(0.,0.,1.));
#10311=DIRECTION('ref_axis',(1.,0.,0.));
#10312=DIRECTION('center_axis',(0.,0.,1.));
#10313=DIRECTION('ref_axis',(1.,0.,0.));
#10314=DIRECTION('center_axis',(0.,0.,1.));
#10315=DIRECTION('ref_axis',(1.,0.,0.));
#10316=DIRECTION('',(0.,0.,1.));
#10317=DIRECTION('center_axis',(0.,0.,1.));
#10318=DIRECTION('ref_axis',(1.,0.,0.));
#10319=DIRECTION('center_axis',(0.,0.,-1.));
#10320=DIRECTION('ref_axis',(-1.,0.,0.));
#10321=DIRECTION('center_axis',(0.,0.,-1.));
#10322=DIRECTION('ref_axis',(1.,0.,0.));
#10323=DIRECTION('center_axis',(0.,0.,1.));
#10324=DIRECTION('ref_axis',(1.,0.,0.));
#10325=DIRECTION('center_axis',(0.,0.,1.));
#10326=DIRECTION('ref_axis',(1.,0.,0.));
#10327=DIRECTION('center_axis',(0.,0.,1.));
#10328=DIRECTION('ref_axis',(1.,0.,0.));
#10329=DIRECTION('center_axis',(0.,0.,1.));
#10330=DIRECTION('ref_axis',(1.,0.,0.));
#10331=DIRECTION('',(0.,0.,-1.));
#10332=DIRECTION('center_axis',(-1.60246890531964E-16,-1.,0.));
#10333=DIRECTION('ref_axis',(1.,-1.60246890531964E-16,0.));
#10334=DIRECTION('',(-1.,1.60246890531964E-16,0.));
#10335=DIRECTION('',(0.,0.,1.));
#10336=DIRECTION('',(1.,-1.60246890531964E-16,0.));
#10337=DIRECTION('',(0.,0.,1.));
#10338=DIRECTION('center_axis',(-0.866025403784439,-0.5,0.));
#10339=DIRECTION('ref_axis',(0.5,-0.866025403784439,0.));
#10340=DIRECTION('',(-0.5,0.866025403784439,0.));
#10341=DIRECTION('',(0.5,-0.866025403784439,0.));
#10342=DIRECTION('',(0.,0.,1.));
#10343=DIRECTION('center_axis',(-0.866025403784439,0.5,0.));
#10344=DIRECTION('ref_axis',(-0.5,-0.866025403784439,0.));
#10345=DIRECTION('',(0.5,0.866025403784439,0.));
#10346=DIRECTION('',(-0.5,-0.866025403784439,0.));
#10347=DIRECTION('',(0.,0.,1.));
#10348=DIRECTION('center_axis',(1.60246890531964E-16,1.,0.));
#10349=DIRECTION('ref_axis',(-1.,1.60246890531964E-16,0.));
#10350=DIRECTION('',(1.,-1.60246890531964E-16,0.));
#10351=DIRECTION('',(-1.,1.60246890531964E-16,0.));
#10352=DIRECTION('',(0.,0.,1.));
#10353=DIRECTION('center_axis',(0.866025403784439,0.5,0.));
#10354=DIRECTION('ref_axis',(-0.5,0.866025403784439,0.));
#10355=DIRECTION('',(0.5,-0.866025403784439,0.));
#10356=DIRECTION('',(-0.5,0.866025403784439,0.));
#10357=DIRECTION('',(0.,0.,1.));
#10358=DIRECTION('center_axis',(0.866025403784439,-0.5,0.));
#10359=DIRECTION('ref_axis',(0.5,0.866025403784439,0.));
#10360=DIRECTION('',(-0.5,-0.866025403784439,0.));
#10361=DIRECTION('',(0.5,0.866025403784439,0.));
#10362=DIRECTION('center_axis',(0.,0.,1.));
#10363=DIRECTION('ref_axis',(1.,0.,0.));
#10364=DIRECTION('center_axis',(0.,0.,1.));
#10365=DIRECTION('ref_axis',(1.,0.,0.));
#10366=DIRECTION('center_axis',(0.,0.,1.));
#10367=DIRECTION('ref_axis',(1.,0.,0.));
#10368=DIRECTION('center_axis',(0.,0.,1.));
#10369=DIRECTION('ref_axis',(1.,0.,0.));
#10370=DIRECTION('center_axis',(0.,0.,1.));
#10371=DIRECTION('ref_axis',(1.,0.,0.));
#10372=DIRECTION('',(0.,0.,-1.));
#10373=DIRECTION('center_axis',(0.,0.,1.));
#10374=DIRECTION('ref_axis',(1.,0.,0.));
#10375=DIRECTION('center_axis',(0.,0.,1.));
#10376=DIRECTION('ref_axis',(1.,0.,0.));
#10377=DIRECTION('center_axis',(0.,0.,1.));
#10378=DIRECTION('ref_axis',(1.,0.,0.));
#10379=DIRECTION('',(0.,0.,-1.));
#10380=DIRECTION('center_axis',(0.,0.,1.));
#10381=DIRECTION('ref_axis',(1.,0.,0.));
#21745=CARTESIAN_POINT('',(0.,0.,0.));
#21746=CARTESIAN_POINT('Origin',(0.,0.,23.));
#21747=CARTESIAN_POINT('',(-1.66862128043148,-0.000391815337284296,18.7714803633902));
#21748=CARTESIAN_POINT('',(-1.66651971410499,0.00146964277546923,18.5785196366098));
#21749=CARTESIAN_POINT('',(-1.666,2.04026156737949E-16,23.));
#21750=CARTESIAN_POINT('',(-0.769902040670449,-1.47743251885542,18.));
#21751=CARTESIAN_POINT('Ctrl Pts',(-1.66651971410499,0.00146964277546923,
18.5785196366098));
#21752=CARTESIAN_POINT('Ctrl Pts',(-1.66756984451206,0.115275174909824,
18.5709016210591));
#21753=CARTESIAN_POINT('Ctrl Pts',(-1.65690316968289,0.228886355259084,
18.5632836055085));
#21754=CARTESIAN_POINT('Ctrl Pts',(-1.63379463140209,0.339911562034265,
18.5556655899578));
#21755=CARTESIAN_POINT('Ctrl Pts',(-1.52142398866744,0.87979745587462,18.5186212172939));
#21756=CARTESIAN_POINT('Ctrl Pts',(-1.1148509467417,1.35853498293726,18.4815768446301));
#21757=CARTESIAN_POINT('Ctrl Pts',(-0.600441280316438,1.55695868566131,
18.4445324719662));
#21758=CARTESIAN_POINT('Ctrl Pts',(-0.0860316138911562,1.75538238838537,
18.4074880993024));
#21759=CARTESIAN_POINT('Ctrl Pts',(0.536214677033665,1.67349226677081,18.3704437266385));
#21760=CARTESIAN_POINT('Ctrl Pts',(0.982144949096516,1.34892973433264,18.3333993539747));
#21761=CARTESIAN_POINT('Ctrl Pts',(1.42807522115936,1.02436720189448,18.2963549813108));
#21762=CARTESIAN_POINT('Ctrl Pts',(1.69768947436024,0.457132258632721,18.259310608647));
#21763=CARTESIAN_POINT('Ctrl Pts',(1.66642050747925,-0.0935369959750123,
18.2222662359831));
#21764=CARTESIAN_POINT('Ctrl Pts',(1.63515154059826,-0.644206250582737,
18.1852218633193));
#21765=CARTESIAN_POINT('Ctrl Pts',(1.30299935363541,-1.17830981653643,18.1481774906554));
#21766=CARTESIAN_POINT('Ctrl Pts',(0.824551049590138,-1.45061632146208,
18.1111331179916));
#21767=CARTESIAN_POINT('Ctrl Pts',(0.346102745544861,-1.72292282638774,
18.0740887453277));
#21768=CARTESIAN_POINT('Ctrl Pts',(-0.278641675582842,-1.73343227028534,
18.0370443726639));
#21769=CARTESIAN_POINT('Ctrl Pts',(-0.769902040670449,-1.47743251885542,
18.));
#21770=CARTESIAN_POINT('',(-1.33705952834865,0.998970281948476,18.));
#21771=CARTESIAN_POINT('Origin',(0.,0.,18.));
#21772=CARTESIAN_POINT('',(-1.66450505821393,-0.00123145023033004,18.0714803633902));
#21773=CARTESIAN_POINT('Ctrl Pts',(-1.33706021092905,0.998970828965241,
18.));
#21774=CARTESIAN_POINT('Ctrl Pts',(-1.54904561011422,0.714506920185143,
18.0238267877967));
#21775=CARTESIAN_POINT('Ctrl Pts',(-1.66218506517322,0.355909860131879,
18.0476535755935));
#21776=CARTESIAN_POINT('Ctrl Pts',(-1.66450505821393,-0.00123145023033004,
18.0714803633902));
#21777=CARTESIAN_POINT('',(-1.666,-2.04026156737949E-16,17.));
#21778=CARTESIAN_POINT('',(-1.666,2.04026156737949E-16,23.));
#21779=CARTESIAN_POINT('Origin',(0.,0.,17.));
#21780=CARTESIAN_POINT('Ctrl Pts',(-1.66450505821393,-0.00123145023033004,
18.0714803633902));
#21781=CARTESIAN_POINT('Ctrl Pts',(-1.66572133056423,-0.188465245039766,
18.0839717212025));
#21782=CARTESIAN_POINT('Ctrl Pts',(-1.63647939540381,-0.3752989338988,18.0964630790149));
#21783=CARTESIAN_POINT('Ctrl Pts',(-1.57505399404498,-0.550840946823039,
18.1089544368272));
#21784=CARTESIAN_POINT('Ctrl Pts',(-1.3928908142571,-1.0714283675521,18.1459988094911));
#21785=CARTESIAN_POINT('Ctrl Pts',(-0.927680991901669,-1.49270793428555,
18.1830431821549));
#21786=CARTESIAN_POINT('Ctrl Pts',(-0.391726107224654,-1.62209767954181,
18.2200875548188));
#21787=CARTESIAN_POINT('Ctrl Pts',(0.144228777452376,-1.75148742479807,
18.2571319274826));
#21788=CARTESIAN_POINT('Ctrl Pts',(0.750928724450993,-1.58898734857712,
18.2941763001465));
#21789=CARTESIAN_POINT('Ctrl Pts',(1.15043245240881,-1.20885486196241,18.3312206728103));
#21790=CARTESIAN_POINT('Ctrl Pts',(1.54993618036662,-0.828722375347701,
18.3682650454742));
#21791=CARTESIAN_POINT('Ctrl Pts',(1.74224368928364,-0.230957478339239,
18.405309418138));
#21792=CARTESIAN_POINT('Ctrl Pts',(1.63950887043352,0.31083583145342,18.4423537908019));
#21793=CARTESIAN_POINT('Ctrl Pts',(1.53677405158339,0.85262914124608,18.4793981634657));
#21794=CARTESIAN_POINT('Ctrl Pts',(1.13899690496613,1.33845086382294,18.5164425361296));
#21795=CARTESIAN_POINT('Ctrl Pts',(0.628126141256631,1.54600803039379,18.5534869087934));
#21796=CARTESIAN_POINT('Ctrl Pts',(0.117255377547129,1.75356519696465,18.5905312814573));
#21797=CARTESIAN_POINT('Ctrl Pts',(-0.506709003254616,1.6828578075295,18.6275756541212));
#21798=CARTESIAN_POINT('Ctrl Pts',(-0.958186006148353,1.36622807375104,
18.664620026785));
#21799=CARTESIAN_POINT('Ctrl Pts',(-1.39230488421667,1.06177193554254,18.7002401389867));
#21800=CARTESIAN_POINT('Ctrl Pts',(-1.66694480132652,0.52994008771394,18.7358602511885));
#21801=CARTESIAN_POINT('Ctrl Pts',(-1.66862128043148,-0.000391815337284296,
18.7714803633902));
#21802=CARTESIAN_POINT('Origin',(0.,0.,23.));
#21803=CARTESIAN_POINT('',(-1.66554933918236,0.00151251337263472,19.4714803633902));
#21804=CARTESIAN_POINT('',(-1.66327374781977,-4.03244713725982E-5,19.2785196366098));
#21805=CARTESIAN_POINT('',(-1.666,2.04026156737949E-16,23.));
#21806=CARTESIAN_POINT('Ctrl Pts',(-1.66327374781977,-4.03244713725982E-5,
19.2785196366098));
#21807=CARTESIAN_POINT('Ctrl Pts',(-1.66321388055115,0.280452962555568,
19.2598345237089));
#21808=CARTESIAN_POINT('Ctrl Pts',(-1.59604427325322,0.560973406431315,
19.241149410808));
#21809=CARTESIAN_POINT('Ctrl Pts',(-1.46192619363535,0.804645854884145,
19.2224642979072));
#21810=CARTESIAN_POINT('Ctrl Pts',(-1.19602894438243,1.28774130291723,19.1854199252433));
#21811=CARTESIAN_POINT('Ctrl Pts',(-0.666987552272445,1.62600395887066,
19.1483755525795));
#21812=CARTESIAN_POINT('Ctrl Pts',(-0.116907900542003,1.66463648121937,
19.1113311799156));
#21813=CARTESIAN_POINT('Ctrl Pts',(0.433171751188448,1.70326900356808,19.0742868072517));
#21814=CARTESIAN_POINT('Ctrl Pts',(1.00428966253935,1.44227139231205,19.0372424345879));
#21815=CARTESIAN_POINT('Ctrl Pts',(1.33510282367111,1.00108454580982,19.000198061924));
#21816=CARTESIAN_POINT('Ctrl Pts',(1.66591598480286,0.559897699307611,18.9631536892602));
#21817=CARTESIAN_POINT('Ctrl Pts',(1.75642439571548,-0.0614783824407909,
18.9261093165963));
#21818=CARTESIAN_POINT('Ctrl Pts',(1.56518696899417,-0.578696033473889,
18.8890649439325));
#21819=CARTESIAN_POINT('Ctrl Pts',(1.37394954227287,-1.09591368450699,18.8520205712686));
#21820=CARTESIAN_POINT('Ctrl Pts',(0.900966277917629,-1.5089729048248,18.8149761986048));
#21821=CARTESIAN_POINT('Ctrl Pts',(0.362727183275646,-1.62883763630031,
18.7779318259409));
#21822=CARTESIAN_POINT('Ctrl Pts',(-0.175511911366353,-1.74870236777582,
18.7408874532771));
#21823=CARTESIAN_POINT('Ctrl Pts',(-0.779006836295083,-1.57537261040905,
18.7038430806132));
#21824=CARTESIAN_POINT('Ctrl Pts',(-1.17167017698769,-1.18819060141662,
18.6667987079494));
#21825=CARTESIAN_POINT('Ctrl Pts',(-1.48358399432579,-0.880630903543001,
18.6373723508362));
#21826=CARTESIAN_POINT('Ctrl Pts',(-1.66246334113382,-0.438130697729091,
18.607945993723));
#21827=CARTESIAN_POINT('Ctrl Pts',(-1.66651971410499,0.00146964277546923,
18.5785196366098));
#21828=CARTESIAN_POINT('Ctrl Pts',(-1.66862128043148,-0.000391815337284296,
18.7714803633902));
#21829=CARTESIAN_POINT('Ctrl Pts',(-1.66868831399082,-0.0215969917005588,
18.7729046238523));
#21830=CARTESIAN_POINT('Ctrl Pts',(-1.6683189395033,-0.042799769984532,
18.7743288843144));
#21831=CARTESIAN_POINT('Ctrl Pts',(-1.66750590227882,-0.0639855189198817,
18.7757531447766));
#21832=CARTESIAN_POINT('Ctrl Pts',(-1.64635917052983,-0.615017299690576,
18.8127975174404));
#21833=CARTESIAN_POINT('Ctrl Pts',(-1.3250760820461,-1.15452878311018,18.8498418901043));
#21834=CARTESIAN_POINT('Ctrl Pts',(-0.850670573251791,-1.43563292242657,
18.8868862627681));
#21835=CARTESIAN_POINT('Ctrl Pts',(-0.376265064457497,-1.71673706174295,
18.923930635432));
#21836=CARTESIAN_POINT('Ctrl Pts',(0.251262864647364,-1.73943385695613,
18.9609750080958));
#21837=CARTESIAN_POINT('Ctrl Pts',(0.74473808845371,-1.49333471419146,18.9980193807597));
#21838=CARTESIAN_POINT('Ctrl Pts',(1.23821331226007,-1.24723557142679,19.0350637534235));
#21839=CARTESIAN_POINT('Ctrl Pts',(1.59763583076791,-0.732340490684249,
19.0721081260874));
#21840=CARTESIAN_POINT('Ctrl Pts',(1.6585299445115,-0.184276682906552,19.1091524987512));
#21841=CARTESIAN_POINT('Ctrl Pts',(1.71942405825509,0.363787124871138,19.1461968714151));
#21842=CARTESIAN_POINT('Ctrl Pts',(1.48178976723445,0.945019659683982,19.1832412440789));
#21843=CARTESIAN_POINT('Ctrl Pts',(1.05437157772921,1.29343804143271,19.2202856167428));
#21844=CARTESIAN_POINT('Ctrl Pts',(0.626953388223968,1.64185642318143,19.2573299894067));
#21845=CARTESIAN_POINT('Ctrl Pts',(0.00975130023412978,1.75746065186603,
19.2943743620705));
#21846=CARTESIAN_POINT('Ctrl Pts',(-0.514790020800312,1.58734766279481,
19.3314187347344));
#21847=CARTESIAN_POINT('Ctrl Pts',(-1.03933134183475,1.41723467372359,19.3684631073982));
#21848=CARTESIAN_POINT('Ctrl Pts',(-1.47121189591379,0.961404466896546,
19.4055074800621));
#21849=CARTESIAN_POINT('Ctrl Pts',(-1.61279508090511,0.428454068820398,
19.4425518527259));
#21850=CARTESIAN_POINT('Ctrl Pts',(-1.64964989746138,0.289724394418121,
19.452194689614));
#21851=CARTESIAN_POINT('Ctrl Pts',(-1.66683453773576,0.145769155066602,
19.4618375265021));
#21852=CARTESIAN_POINT('Ctrl Pts',(-1.66554933918236,0.00151251337263472,
19.4714803633902));
#21853=CARTESIAN_POINT('Origin',(0.,0.,23.));
#21854=CARTESIAN_POINT('',(-1.66342907320707,-0.00052814431987333,20.1714803633902));
#21855=CARTESIAN_POINT('',(-1.66660945832472,-0.0014645595731799,19.9785196366098));
#21856=CARTESIAN_POINT('',(-1.666,2.04026156737949E-16,23.));
#21857=CARTESIAN_POINT('Ctrl Pts',(-1.66660945832472,-0.0014645595731799,
19.9785196366098));
#21858=CARTESIAN_POINT('Ctrl Pts',(-1.66253083892564,0.442903547938621,
19.9487674263587));
#21859=CARTESIAN_POINT('Ctrl Pts',(-1.47929031344958,0.890241199679583,
19.9190152161076));
#21860=CARTESIAN_POINT('Ctrl Pts',(-1.16122364049601,1.19843253381782,19.8892630058565));
#21861=CARTESIAN_POINT('Ctrl Pts',(-0.765199941234552,1.58216048334607,
19.8522186331927));
#21862=CARTESIAN_POINT('Ctrl Pts',(-0.160159946883716,1.75017472804193,
19.8151742605288));
#21863=CARTESIAN_POINT('Ctrl Pts',(0.377018012610026,1.62558860949911,19.778129887865));
#21864=CARTESIAN_POINT('Ctrl Pts',(0.914195972103768,1.50100249095629,19.7410855152011));
#21865=CARTESIAN_POINT('Ctrl Pts',(1.38351189674041,1.08381600917481,19.7040411425372));
#21866=CARTESIAN_POINT('Ctrl Pts',(1.57019781685605,0.564941972855801,19.6669967698734));
#21867=CARTESIAN_POINT('Ctrl Pts',(1.75688373697169,0.0460679365367972,
19.6299523972095));
#21868=CARTESIAN_POINT('Ctrl Pts',(1.66093965256632,-0.574493654319738,
19.5929080245457));
#21869=CARTESIAN_POINT('Ctrl Pts',(1.32627101594693,-1.01276172717728,19.5558636518818));
#21870=CARTESIAN_POINT('Ctrl Pts',(0.991602379327531,-1.45102980003482,
19.518819279218));
#21871=CARTESIAN_POINT('Ctrl Pts',(0.418209190494114,-1.70700435489339,
19.4817749065541));
#21872=CARTESIAN_POINT('Ctrl Pts',(-0.131511680146043,-1.66354615959309,
19.4447305338903));
#21873=CARTESIAN_POINT('Ctrl Pts',(-0.681232550786199,-1.62008796429278,
19.4076861612264));
#21874=CARTESIAN_POINT('Ctrl Pts',(-1.20728110323309,-1.27719701883361,
19.3706417885626));
#21875=CARTESIAN_POINT('Ctrl Pts',(-1.46892882625861,-0.791787426047646,
19.3335974158987));
#21876=CARTESIAN_POINT('Ctrl Pts',(-1.59860192281783,-0.551217532038033,
19.3152381561358));
#21877=CARTESIAN_POINT('Ctrl Pts',(-1.66333257105202,-0.275642037215341,
19.2968788963728));
#21878=CARTESIAN_POINT('Ctrl Pts',(-1.66327374781977,-4.03244713725982E-5,
19.2785196366098));
#21879=CARTESIAN_POINT('Ctrl Pts',(-1.66554933918236,0.00151251337263472,
19.4714803633902));
#21880=CARTESIAN_POINT('Ctrl Pts',(-1.66189725893372,-0.408413898754999,
19.498881899166));
#21881=CARTESIAN_POINT('Ctrl Pts',(-1.50910204174448,-0.820774121553807,
19.5262834349417));
#21882=CARTESIAN_POINT('Ctrl Pts',(-1.23470683773252,-1.12257747109454,
19.5536849707175));
#21883=CARTESIAN_POINT('Ctrl Pts',(-0.863749593664997,-1.53058802360804,
19.5907293433813));
#21884=CARTESIAN_POINT('Ctrl Pts',(-0.27054928962637,-1.73653853930977,
19.6277737160452));
#21885=CARTESIAN_POINT('Ctrl Pts',(0.27343382250233,-1.64618196770234,19.664818088709));
#21886=CARTESIAN_POINT('Ctrl Pts',(0.817416934631023,-1.55582539609492,
19.7018624613729));
#21887=CARTESIAN_POINT('Ctrl Pts',(1.31218285484979,-1.16916173717834,19.7389068340367));
#21888=CARTESIAN_POINT('Ctrl Pts',(1.53131702289696,-0.663135912295698,
19.7759512067006));
#21889=CARTESIAN_POINT('Ctrl Pts',(1.75045119094414,-0.157110087413051,
19.8129955793645));
#21890=CARTESIAN_POINT('Ctrl Pts',(1.69395360681972,0.46827790343567,19.8500399520283));
#21891=CARTESIAN_POINT('Ctrl Pts',(1.38767864477499,0.92683821933391,19.8870843246922));
#21892=CARTESIAN_POINT('Ctrl Pts',(1.08140368273026,1.38539853523215,19.924128697356));
#21893=CARTESIAN_POINT('Ctrl Pts',(0.525351342765218,1.67713117617991,19.9611730700199));
#21894=CARTESIAN_POINT('Ctrl Pts',(-0.0260178646503011,1.66853353860585,
19.9982174426837));
#21895=CARTESIAN_POINT('Ctrl Pts',(-0.577387072065821,1.6599359010318,20.0352618153476));
#21896=CARTESIAN_POINT('Ctrl Pts',(-1.12407314693182,1.35100798493592,20.0723061880114));
#21897=CARTESIAN_POINT('Ctrl Pts',(-1.41590179139748,0.883121287398709,
20.1093505606753));
#21898=CARTESIAN_POINT('Ctrl Pts',(-1.5790507827593,0.621545721660193,20.1300604949136));
#21899=CARTESIAN_POINT('Ctrl Pts',(-1.66254528607668,0.31028833838162,20.1507704291519));
#21900=CARTESIAN_POINT('Ctrl Pts',(-1.66342907320707,-0.00052814431987333,
20.1714803633902));
#21901=CARTESIAN_POINT('Origin',(0.,0.,23.));
#21902=CARTESIAN_POINT('',(-1.6674840545265,-0.00123301224869695,20.8714803633902));
#21903=CARTESIAN_POINT('',(-1.66803766879579,0.000959062403117482,20.6785196366098));
#21904=CARTESIAN_POINT('',(-1.666,2.04026156737949E-16,23.));
#21905=CARTESIAN_POINT('Ctrl Pts',(-1.66803766879579,0.000959062403117482,
20.6785196366098));
#21906=CARTESIAN_POINT('Ctrl Pts',(-1.66842376314776,0.0572146414461489,
20.6747447016723));
#21907=CARTESIAN_POINT('Ctrl Pts',(-1.66582448293573,0.113434120530944,
20.6709697667349));
#21908=CARTESIAN_POINT('Ctrl Pts',(-1.66012222476806,0.169337087226355,
20.6671948317974));
#21909=CARTESIAN_POINT('Ctrl Pts',(-1.60416455130123,0.71792676243648,20.6301504591336));
#21910=CARTESIAN_POINT('Ctrl Pts',(-1.24939060962216,1.23603634645977,20.5931060864697));
#21911=CARTESIAN_POINT('Ctrl Pts',(-0.758151936074614,1.48656869769561,
20.5560617138059));
#21912=CARTESIAN_POINT('Ctrl Pts',(-0.266913262527071,1.73710104893144,
20.519017341142));
#21913=CARTESIAN_POINT('Ctrl Pts',(0.360790142888952,1.72005616737984,20.4819729684781));
#21914=CARTESIAN_POINT('Ctrl Pts',(0.837708846366109,1.44323412561422,20.4449285958143));
#21915=CARTESIAN_POINT('Ctrl Pts',(1.31462754984327,1.1664120838486,20.4078842231504));
#21916=CARTESIAN_POINT('Ctrl Pts',(1.64076155138155,0.629812881868986,20.3708398504866));
#21917=CARTESIAN_POINT('Ctrl Pts',(1.66686551824842,0.0789948759482206,
20.3337954778227));
#21918=CARTESIAN_POINT('Ctrl Pts',(1.69296948511529,-0.471823129972545,
20.2967511051589));
#21919=CARTESIAN_POINT('Ctrl Pts',(1.4190434173107,-1.03685993983447,20.259706732495));
#21920=CARTESIAN_POINT('Ctrl Pts',(0.970441265381544,-1.35754359208473,
20.2226623598312));
#21921=CARTESIAN_POINT('Ctrl Pts',(0.521839113452374,-1.67822724433501,
20.1856179871673));
#21922=CARTESIAN_POINT('Ctrl Pts',(-0.101439122601358,-1.75455773897363,
20.1485736145035));
#21923=CARTESIAN_POINT('Ctrl Pts',(-0.614169038869319,-1.55160473476285,
20.1115292418396));
#21924=CARTESIAN_POINT('Ctrl Pts',(-1.12689895513726,-1.34865173055207,
20.0744848691758));
#21925=CARTESIAN_POINT('Ctrl Pts',(-1.52908055161943,-0.866415227491897,
20.0374404965119));
#21926=CARTESIAN_POINT('Ctrl Pts',(-1.63666764777447,-0.325576148781487,
20.0003961238481));
#21927=CARTESIAN_POINT('Ctrl Pts',(-1.65784610275328,-0.219112302385464,
19.9931039614353));
#21928=CARTESIAN_POINT('Ctrl Pts',(-1.66760911363862,-0.1103776246422,19.9858117990225));
#21929=CARTESIAN_POINT('Ctrl Pts',(-1.66660945832472,-0.0014645595731799,
19.9785196366098));
#21930=CARTESIAN_POINT('Ctrl Pts',(-1.66342907320707,-0.00052814431987333,
20.1714803633902));
#21931=CARTESIAN_POINT('Ctrl Pts',(-1.66412613802131,-0.24567680775405,
20.1878148018158));
#21932=CARTESIAN_POINT('Ctrl Pts',(-1.61343216789926,-0.490551192765208,
20.2041492402413));
#21933=CARTESIAN_POINT('Ctrl Pts',(-1.50989667393363,-0.710558323734967,
20.2204836786668));
#21934=CARTESIAN_POINT('Ctrl Pts',(-1.2750916979388,-1.20950575835288,20.2575280513307));
#21935=CARTESIAN_POINT('Ctrl Pts',(-0.768510531883807,-1.58055514861014,
20.2945724239946));
#21936=CARTESIAN_POINT('Ctrl Pts',(-0.221974689125013,-1.65390699052376,
20.3316167966584));
#21937=CARTESIAN_POINT('Ctrl Pts',(0.324561153633781,-1.72725883243739,
20.3686611693222));
#21938=CARTESIAN_POINT('Ctrl Pts',(0.911051673096376,-1.50291312600738,
20.4057055419861));
#21939=CARTESIAN_POINT('Ctrl Pts',(1.26910726675768,-1.08353488200329,20.4427499146499));
#21940=CARTESIAN_POINT('Ctrl Pts',(1.62716286041898,-0.664156637999206,
20.4797942873138));
#21941=CARTESIAN_POINT('Ctrl Pts',(1.75678352827899,-0.0497458564210427,
20.5168386599777));
#21942=CARTESIAN_POINT('Ctrl Pts',(1.59865230117954,0.478530997816609,20.5538830326415));
#21943=CARTESIAN_POINT('Ctrl Pts',(1.44052107408009,1.00680785205427,20.5909274053054));
#21944=CARTESIAN_POINT('Ctrl Pts',(0.994637952021168,1.44895077895141,20.6279717779692));
#21945=CARTESIAN_POINT('Ctrl Pts',(0.46504782688183,1.60262647375647,20.6650161506331));
#21946=CARTESIAN_POINT('Ctrl Pts',(-0.0645422982574929,1.75630216856152,
20.7020605232969));
#21947=CARTESIAN_POINT('Ctrl Pts',(-0.677839426477227,1.62151063127449,
20.7391048959608));
#21948=CARTESIAN_POINT('Ctrl Pts',(-1.09418672250608,1.25993512208958,20.7761492686246));
#21949=CARTESIAN_POINT('Ctrl Pts',(-1.45133357711098,0.949772051404937,
20.8079263002132));
#21950=CARTESIAN_POINT('Ctrl Pts',(-1.6635572776099,0.472732735422094,20.8397033318017));
#21951=CARTESIAN_POINT('Ctrl Pts',(-1.6674840545265,-0.00123301224869695,
20.8714803633902));
#21952=CARTESIAN_POINT('Origin',(0.,0.,23.));
#21953=CARTESIAN_POINT('',(-1.66726411708323,0.00131035561855258,21.5714803633902));
#21954=CARTESIAN_POINT('',(-1.66370962959227,0.000855487351938633,21.3785196366098));
#21955=CARTESIAN_POINT('',(-1.666,2.04026156737949E-16,23.));
#21956=CARTESIAN_POINT('Ctrl Pts',(-1.66370962959227,0.000855487351938633,
21.3785196366098));
#21957=CARTESIAN_POINT('Ctrl Pts',(-1.66474566899998,0.223512053075316,
21.3636776043221));
#21958=CARTESIAN_POINT('Ctrl Pts',(-1.62319372826002,0.445797790127472,
21.3488355720344));
#21959=CARTESIAN_POINT('Ctrl Pts',(-1.53722532564539,0.649322068833036,
21.3339935397468));
#21960=CARTESIAN_POINT('Ctrl Pts',(-1.32265595387433,1.15730029448153,21.2969491670829));
#21961=CARTESIAN_POINT('Ctrl Pts',(-0.83139133092368,1.54840278958771,21.2599047944191));
#21962=CARTESIAN_POINT('Ctrl Pts',(-0.288243816224439,1.64365335557573,
21.2228604217552));
#21963=CARTESIAN_POINT('Ctrl Pts',(0.254903698474809,1.73890392156375,21.1858160490914));
#21964=CARTESIAN_POINT('Ctrl Pts',(0.849934104922654,1.53830255843362,21.1487716764275));
#21965=CARTESIAN_POINT('Ctrl Pts',(1.22454977899659,1.13364839773686,21.1117273037637));
#21966=CARTESIAN_POINT('Ctrl Pts',(1.59916545307052,0.728994237040111,21.0746829310998));
#21967=CARTESIAN_POINT('Ctrl Pts',(1.75336639477056,0.120287278776759,21.037638558436));
#21968=CARTESIAN_POINT('Ctrl Pts',(1.61658721862146,-0.413916193690381,
21.0005941857721));
#21969=CARTESIAN_POINT('Ctrl Pts',(1.47980804247235,-0.948119666157537,
20.9635498131082));
#21970=CARTESIAN_POINT('Ctrl Pts',(1.05204874847409,-1.40781965282848,20.9265054404444));
#21971=CARTESIAN_POINT('Ctrl Pts',(0.529060407604963,-1.58264839304365,
20.8894610677805));
#21972=CARTESIAN_POINT('Ctrl Pts',(0.00607206673584673,-1.75747713325882,
20.8524166951167));
#21973=CARTESIAN_POINT('Ctrl Pts',(-0.612145321004125,-1.64743462701824,
20.8153723224528));
#21974=CARTESIAN_POINT('Ctrl Pts',(-1.04268331224681,-1.30287849069947,
20.778327949789));
#21975=CARTESIAN_POINT('Ctrl Pts',(-1.42934816465156,-0.993433679080626,
20.7450585120626));
#21976=CARTESIAN_POINT('Ctrl Pts',(-1.66463492352674,-0.494835306173304,
20.7117890743362));
#21977=CARTESIAN_POINT('Ctrl Pts',(-1.66803766879579,0.000959062403117482,
20.6785196366098));
#21978=CARTESIAN_POINT('Ctrl Pts',(-1.6674840545265,-0.00123301224869695,
20.8714803633902));
#21979=CARTESIAN_POINT('Ctrl Pts',(-1.66813495463619,-0.0797972810366568,
20.8767477044655));
#21980=CARTESIAN_POINT('Ctrl Pts',(-1.6630626525888,-0.15827709993217,20.8820150455409));
#21981=CARTESIAN_POINT('Ctrl Pts',(-1.65197851677833,-0.235898443844886,
20.8872823866162));
#21982=CARTESIAN_POINT('Ctrl Pts',(-1.57402555118372,-0.78179701951157,
20.92432675928));
#21983=CARTESIAN_POINT('Ctrl Pts',(-1.19872215615655,-1.28523468976212,
20.9613711319439));
#21984=CARTESIAN_POINT('Ctrl Pts',(-0.697814551206597,-1.51582846911685,
20.9984155046078));
#21985=CARTESIAN_POINT('Ctrl Pts',(-0.196906946256626,-1.74642224847158,
21.0354598772716));
#21986=CARTESIAN_POINT('Ctrl Pts',(0.429604868616143,-1.70417213693048,
21.0725042499355));
#21987=CARTESIAN_POINT('Ctrl Pts',(0.895016757317744,-1.40841261701728,
21.1095486225993));
#21988=CARTESIAN_POINT('Ctrl Pts',(1.36042864601934,-1.11265309710409,21.1465929952632));
#21989=CARTESIAN_POINT('Ctrl Pts',(1.66474060854977,-0.563384168818808,
21.183637367927));
#21990=CARTESIAN_POINT('Ctrl Pts',(1.66869350204147,-0.0119621032475723,
21.2206817405909));
#21991=CARTESIAN_POINT('Ctrl Pts',(1.67264639553316,0.539459962323664,21.2577261132547));
#21992=CARTESIAN_POINT('Ctrl Pts',(1.37624021998613,1.09303516518086,21.2947704859186));
#21993=CARTESIAN_POINT('Ctrl Pts',(0.915116274553919,1.39543659824045,21.3318148585824));
#21994=CARTESIAN_POINT('Ctrl Pts',(0.453992329121703,1.69783803130004,21.3688592312463));
#21995=CARTESIAN_POINT('Ctrl Pts',(-0.171849386195692,1.74906569456202,
21.4059036039101));
#21996=CARTESIAN_POINT('Ctrl Pts',(-0.676011386027486,1.52567680116829,
21.442947976574));
#21997=CARTESIAN_POINT('Ctrl Pts',(-1.18017338585927,1.30228790777458,21.4799923492378));
#21998=CARTESIAN_POINT('Ctrl Pts',(-1.56265567020546,0.804282457725167,
21.5170367219017));
#21999=CARTESIAN_POINT('Ctrl Pts',(-1.64842681856946,0.259557545613813,
21.5540810945656));
#22000=CARTESIAN_POINT('Ctrl Pts',(-1.66185535629751,0.174274100385222,
21.5598808508404));
#22001=CARTESIAN_POINT('Ctrl Pts',(-1.668010973462,0.0878454775911748,21.5656806071153));
#22002=CARTESIAN_POINT('Ctrl Pts',(-1.66726411708323,0.00131035561855258,
21.5714803633902));
#22003=CARTESIAN_POINT('Origin',(0.,0.,23.));
#22004=CARTESIAN_POINT('',(-1.66336233325601,0.000403110553041652,22.2714803633902));
#22005=CARTESIAN_POINT('',(-1.66491696675796,-0.00142189824448361,22.0785196366098));
#22006=CARTESIAN_POINT('',(-1.666,2.04026156737949E-16,23.));
#22007=CARTESIAN_POINT('Ctrl Pts',(-1.66491696675796,-0.00142189824448361,
22.0785196366098));
#22008=CARTESIAN_POINT('Ctrl Pts',(-1.6617648131379,0.386551789612628,22.0526105069719));
#22009=CARTESIAN_POINT('Ctrl Pts',(-1.52658714042526,0.776505475615136,
22.026701377334));
#22010=CARTESIAN_POINT('Ctrl Pts',(-1.27881118667522,1.07206473672234,22.0007922476961));
#22011=CARTESIAN_POINT('Ctrl Pts',(-0.924545918171753,1.49464965430663,
21.9637478750323));
#22012=CARTESIAN_POINT('Ctrl Pts',(-0.340099051292463,1.72426662069324,
21.9267035023684));
#22013=CARTESIAN_POINT('Ctrl Pts',(0.207075025876924,1.65583839324593,21.8896591297046));
#22014=CARTESIAN_POINT('Ctrl Pts',(0.75424910304631,1.58741016579862,21.8526147570407));
#22015=CARTESIAN_POINT('Ctrl Pts',(1.26415039050579,1.22093674451738,21.8155703843769));
#22016=CARTESIAN_POINT('Ctrl Pts',(1.50343802435341,0.724123579106914,21.778526011713));
#22017=CARTESIAN_POINT('Ctrl Pts',(1.74272565820104,0.227310413696437,21.7414816390492));
#22018=CARTESIAN_POINT('Ctrl Pts',(1.7113996384368,-0.399842495843283,21.7044372663853));
#22019=CARTESIAN_POINT('Ctrl Pts',(1.42379536819668,-0.870337635857372,
21.6673928937215));
#22020=CARTESIAN_POINT('Ctrl Pts',(1.13619109795657,-1.34083277587145,21.6303485210576));
#22021=CARTESIAN_POINT('Ctrl Pts',(0.592308577240593,-1.65467014635991,
21.5933041483937));
#22022=CARTESIAN_POINT('Ctrl Pts',(0.0410391510285976,-1.66823159032892,
21.5562597757299));
#22023=CARTESIAN_POINT('Ctrl Pts',(-0.510230275183399,-1.68179303429794,
21.519215403066));
#22024=CARTESIAN_POINT('Ctrl Pts',(-1.06888660689141,-1.3950785517475,21.4821710304022));
#22025=CARTESIAN_POINT('Ctrl Pts',(-1.37927771244968,-0.939294332376885,
21.4451266577383));
#22026=CARTESIAN_POINT('Ctrl Pts',(-1.5653089090872,-0.666122575133674,
21.4229243173622));
#22027=CARTESIAN_POINT('Ctrl Pts',(-1.6621598081711,-0.332218633722869,
21.400721976986));
#22028=CARTESIAN_POINT('Ctrl Pts',(-1.66370962959227,0.000855487351938633,
21.3785196366098));
#22029=CARTESIAN_POINT('Ctrl Pts',(-1.66726411708323,0.00131035561855258,
21.5714803633902));
#22030=CARTESIAN_POINT('Ctrl Pts',(-1.66324063058717,-0.46487418077553,
21.6027249797792));
#22031=CARTESIAN_POINT('Ctrl Pts',(-1.45889191058994,-0.93414956173162,
21.6339695961681));
#22032=CARTESIAN_POINT('Ctrl Pts',(-1.11213714530839,-1.2441189917722,21.6652142125571));
#22033=CARTESIAN_POINT('Ctrl Pts',(-0.701016311301517,-1.61162624287356,
21.7022585852209));
#22034=CARTESIAN_POINT('Ctrl Pts',(-0.0897146309059634,-1.75519637090299,
21.7393029578848));
#22035=CARTESIAN_POINT('Ctrl Pts',(0.442024216629908,-1.60912885984179,
21.7763473305487));
#22036=CARTESIAN_POINT('Ctrl Pts',(0.973763064165779,-1.46306134878059,
21.8133917032125));
#22037=CARTESIAN_POINT('Ctrl Pts',(1.42593907884196,-1.02735619862877,21.8504360758764));
#22038=CARTESIAN_POINT('Ctrl Pts',(1.59162761760514,-0.501400660689515,
21.8874804485402));
#22039=CARTESIAN_POINT('Ctrl Pts',(1.75731615636832,0.02455487724974,21.9245248212041));
#22040=CARTESIAN_POINT('Ctrl Pts',(1.63651721921848,0.64076080297644,21.9615691938679));
#22041=CARTESIAN_POINT('Ctrl Pts',(1.28451077709545,1.06522915806354,21.9986135665318));
#22042=CARTESIAN_POINT('Ctrl Pts',(0.93250433497242,1.48969751315065,22.0356579391956));
#22043=CARTESIAN_POINT('Ctrl Pts',(0.34929038787619,1.72242829759816,22.0727023118595));
#22044=CARTESIAN_POINT('Ctrl Pts',(-0.19824088446344,1.65691932434573,22.1097466845233));
#22045=CARTESIAN_POINT('Ctrl Pts',(-0.745772156803077,1.59141035109329,
22.1467910571872));
#22046=CARTESIAN_POINT('Ctrl Pts',(-1.25762075438611,1.22766162014088,22.183835429851));
#22047=CARTESIAN_POINT('Ctrl Pts',(-1.49955468587626,0.732131709277595,
22.2208798025149));
#22048=CARTESIAN_POINT('Ctrl Pts',(-1.60971080179752,0.506509573650329,
22.23774665614));
#22049=CARTESIAN_POINT('Ctrl Pts',(-1.66391046875662,0.253567667020629,
22.2546135097651));
#22050=CARTESIAN_POINT('Ctrl Pts',(-1.66336233325601,0.000403110553041652,
22.2714803633902));
#22051=CARTESIAN_POINT('Origin',(0.,0.,23.));
#22052=CARTESIAN_POINT('',(-1.66578620297286,-0.00152257679421897,22.9714803633902));
#22053=CARTESIAN_POINT('',(-1.66873613391169,-1.89540107977907E-5,22.7785196366098));
#22054=CARTESIAN_POINT('',(-1.666,2.04026156737949E-16,23.));
#22055=CARTESIAN_POINT('Ctrl Pts',(-1.66873602989402,-1.89532902365601E-5,
22.7785196366098));
#22056=CARTESIAN_POINT('Ctrl Pts',(-1.66864347242946,0.550403095397029,
22.7415434096217));
#22057=CARTESIAN_POINT('Ctrl Pts',(-1.36953979702872,1.10091133072281,22.7045671826336));
#22058=CARTESIAN_POINT('Ctrl Pts',(-0.907660834486349,1.40029734714771,
22.6675909556455));
#22059=CARTESIAN_POINT('Ctrl Pts',(-0.444930647885177,1.70023511977004,
22.6305465829816));
#22060=CARTESIAN_POINT('Ctrl Pts',(0.181175355132312,1.74812420457462,22.5935022103178));
#22061=CARTESIAN_POINT('Ctrl Pts',(0.684138745939249,1.52204961390686,22.5564578376539));
#22062=CARTESIAN_POINT('Ctrl Pts',(1.1871021367462,1.2959750232391,22.51941346499));
#22063=CARTESIAN_POINT('Ctrl Pts',(1.56692291534261,0.795936757098989,22.4823690923262));
#22064=CARTESIAN_POINT('Ctrl Pts',(1.64978761864264,0.250762166729425,22.4453247196624));
#22065=CARTESIAN_POINT('Ctrl Pts',(1.73265232194267,-0.294412423640124,
22.4082803469985));
#22066=CARTESIAN_POINT('Ctrl Pts',(1.51856094994635,-0.88472333823912,22.3712359743346));
#22067=CARTESIAN_POINT('Ctrl Pts',(1.10548592775637,-1.25003268534147,22.3341916016708));
#22068=CARTESIAN_POINT('Ctrl Pts',(0.692410905566374,-1.61534203244382,
22.2971472290069));
#22069=CARTESIAN_POINT('Ctrl Pts',(0.0803522331827074,-1.75564981204952,
22.2601028563431));
#22070=CARTESIAN_POINT('Ctrl Pts',(-0.450599995714626,-1.60674842298081,
22.2230584836792));
#22071=CARTESIAN_POINT('Ctrl Pts',(-0.981552224611956,-1.4578470339121,
22.1860141110154));
#22072=CARTESIAN_POINT('Ctrl Pts',(-1.43139801002296,-1.01973647616899,
22.1489697383515));
#22073=CARTESIAN_POINT('Ctrl Pts',(-1.59427906766464,-0.492904762906453,
22.1119253656877));
#22074=CARTESIAN_POINT('Ctrl Pts',(-1.64323981475635,-0.334543350926403,
22.1007901226617));
#22075=CARTESIAN_POINT('Ctrl Pts',(-1.66627170144435,-0.168165488721959,
22.0896548796358));
#22076=CARTESIAN_POINT('Ctrl Pts',(-1.66491696675796,-0.00142189824448361,
22.0785196366098));
#22077=CARTESIAN_POINT('Ctrl Pts',(-1.66336233325601,0.000403110553041652,
22.2714803633902));
#22078=CARTESIAN_POINT('Ctrl Pts',(-1.66270660843943,-0.302453176197396,
22.291657882429));
#22079=CARTESIAN_POINT('Ctrl Pts',(-1.58370177298327,-0.605628095221617,
22.3118354014677));
#22080=CARTESIAN_POINT('Ctrl Pts',(-1.42841701687781,-0.862731662544646,
22.3320129205065));
#22081=CARTESIAN_POINT('Ctrl Pts',(-1.14332615099193,-1.33475403272947,
22.3690572931703));
#22082=CARTESIAN_POINT('Ctrl Pts',(-0.601125153822886,-1.65148768232495,
22.4061016658342));
#22083=CARTESIAN_POINT('Ctrl Pts',(-0.0499358720868693,-1.6679890600187,
22.443146038498));
#22084=CARTESIAN_POINT('Ctrl Pts',(0.501253409649147,-1.68449043771246,
22.4801904111619));
#22085=CARTESIAN_POINT('Ctrl Pts',(1.06143097595213,-1.4007595435045,22.5172347838257));
#22086=CARTESIAN_POINT('Ctrl Pts',(1.37424854829476,-0.946637218353961,
22.5542791564896));
#22087=CARTESIAN_POINT('Ctrl Pts',(1.68706612063737,-0.492514893203437,
22.5913235291534));
#22088=CARTESIAN_POINT('Ctrl Pts',(1.75252369901963,0.131998862889646,22.6283679018173));
#22089=CARTESIAN_POINT('Ctrl Pts',(1.54066660738123,0.641114264826145,22.6654122744811));
#22090=CARTESIAN_POINT('Ctrl Pts',(1.32880951574283,1.15022966676265,22.702456647145));
#22091=CARTESIAN_POINT('Ctrl Pts',(0.839637754083762,1.54394671454257,22.7395010198089));
#22092=CARTESIAN_POINT('Ctrl Pts',(0.297005947345673,1.64209273882581,22.7765453924727));
#22093=CARTESIAN_POINT('Ctrl Pts',(-0.245625859392417,1.74023876310906,
22.8135897651366));
#22094=CARTESIAN_POINT('Ctrl Pts',(-0.841717711209527,1.54281376389563,
22.8506341378004));
#22095=CARTESIAN_POINT('Ctrl Pts',(-1.21848624574082,1.14016330611172,22.8876785104643));
#22096=CARTESIAN_POINT('Ctrl Pts',(-1.50259508645847,0.836537752779009,
22.9156124614396));
#22097=CARTESIAN_POINT('Ctrl Pts',(-1.66199284431962,0.416217406185016,
22.9435464124149));
#22098=CARTESIAN_POINT('Ctrl Pts',(-1.66578620297286,-0.00152257679421897,
22.9714803633902));
#22099=CARTESIAN_POINT('Origin',(0.,0.,23.));
#22100=CARTESIAN_POINT('',(-1.66853019577507,0.000530614451512978,23.6714803633902));
#22101=CARTESIAN_POINT('',(-1.66497222359982,0.00143386426241622,23.4785196366098));
#22102=CARTESIAN_POINT('',(-1.666,2.04026156737949E-16,23.));
#22103=CARTESIAN_POINT('Ctrl Pts',(-1.66497222359982,0.00143386426241622,
23.4785196366098));
#22104=CARTESIAN_POINT('Ctrl Pts',(-1.66632491173626,0.16612274283444,23.4675206849353));
#22105=CARTESIAN_POINT('Ctrl Pts',(-1.64386439031773,0.330450820220333,
23.4565217332608));
#22106=CARTESIAN_POINT('Ctrl Pts',(-1.59607730938674,0.487050380710409,
23.4455227815864));
#22107=CARTESIAN_POINT('Ctrl Pts',(-1.4351308404033,1.01447632542622,23.4084784089225));
#22108=CARTESIAN_POINT('Ctrl Pts',(-0.986895966349284,1.45423488320508,
23.3714340362587));
#22109=CARTESIAN_POINT('Ctrl Pts',(-0.45649378676817,1.60508388364329,23.3343896635948));
#22110=CARTESIAN_POINT('Ctrl Pts',(0.073908392812964,1.75593288408151,23.297345290931));
#22111=CARTESIAN_POINT('Ctrl Pts',(0.686477877921196,1.61787232717907,23.2603009182671));
#22112=CARTESIAN_POINT('Ctrl Pts',(1.10089081692101,1.25408144077981,23.2232565456033));
#22113=CARTESIAN_POINT('Ctrl Pts',(1.51530375592082,0.890290554380557,23.1862121729394));
#22114=CARTESIAN_POINT('Ctrl Pts',(1.73156014881221,0.300769338484503,23.1491678002756));
#22115=CARTESIAN_POINT('Ctrl Pts',(1.65069681432376,-0.244705696849849,
23.1121234276117));
#22116=CARTESIAN_POINT('Ctrl Pts',(1.5698334798353,-0.790180732184218,23.0750790549479));
#22117=CARTESIAN_POINT('Ctrl Pts',(1.19185041796697,-1.29160958695689,23.038034682284));
#22118=CARTESIAN_POINT('Ctrl Pts',(0.689720116463903,-1.51952854920018,
23.0009903096202));
#22119=CARTESIAN_POINT('Ctrl Pts',(0.187589814960836,-1.74744751144346,
22.9639459369563));
#22120=CARTESIAN_POINT('Ctrl Pts',(-0.438687726176967,-1.70185658115737,
22.9269015642925));
#22121=CARTESIAN_POINT('Ctrl Pts',(-0.902515579102954,-1.40361906526159,
22.8898571916286));
#22122=CARTESIAN_POINT('Ctrl Pts',(-1.36719667532058,-1.10483292090776,
22.852744673289));
#22123=CARTESIAN_POINT('Ctrl Pts',(-1.66882892851784,-0.552469812676142,
22.8156321549494));
#22124=CARTESIAN_POINT('Ctrl Pts',(-1.66873602989402,-1.89532902365601E-5,
22.7785196366098));
#22125=CARTESIAN_POINT('Ctrl Pts',(-1.66578620297286,-0.00152257679421897,
22.9714803633902));
#22126=CARTESIAN_POINT('Ctrl Pts',(-1.66702337479211,-0.137764936654608,
22.9805907850788));
#22127=CARTESIAN_POINT('Ctrl Pts',(-1.6517091709214,-0.273732827619376,
22.9897012067673));
#22128=CARTESIAN_POINT('Ctrl Pts',(-1.61877186757403,-0.405288460746241,
22.9988116284558));
#22129=CARTESIAN_POINT('Ctrl Pts',(-1.48484373763047,-0.9402138534659,23.0358560011197));
#22130=CARTESIAN_POINT('Ctrl Pts',(-1.05954226049788,-1.40218872255081,
23.0729003737835));
#22131=CARTESIAN_POINT('Ctrl Pts',(-0.537493761963633,-1.57980427633088,
23.1099447464474));
#22132=CARTESIAN_POINT('Ctrl Pts',(-0.0154452634293974,-1.75741983011095,
23.1469891191112));
#22133=CARTESIAN_POINT('Ctrl Pts',(0.603350256506486,-1.65067606858619,
23.1840334917751));
#22134=CARTESIAN_POINT('Ctrl Pts',(1.03571979014419,-1.30842103772709,23.2210778644389));
#22135=CARTESIAN_POINT('Ctrl Pts',(1.46808932378189,-0.966166006867992,
23.2581222371028));
#22136=CARTESIAN_POINT('Ctrl Pts',(1.71403287112142,-0.388399706674552,
23.2951666097666));
#22137=CARTESIAN_POINT('Ctrl Pts',(1.66100182477836,0.160480633554725,23.3322109824305));
#22138=CARTESIAN_POINT('Ctrl Pts',(1.6079707784353,0.709360973784014,23.3692553550943));
#22139=CARTESIAN_POINT('Ctrl Pts',(1.25596513840964,1.22935535404913,23.4062997277582));
#22140=CARTESIAN_POINT('Ctrl Pts',(0.766069612980623,1.48250411255109,23.4433441004221));
#22141=CARTESIAN_POINT('Ctrl Pts',(0.276174087551608,1.73565287105304,23.4803884730859));
#22142=CARTESIAN_POINT('Ctrl Pts',(-0.351611323280771,1.72195600779182,
23.5174328457498));
#22143=CARTESIAN_POINT('Ctrl Pts',(-0.82999966082312,1.44768147694742,23.5544772184136));
#22144=CARTESIAN_POINT('Ctrl Pts',(-1.30838799836547,1.17340694610302,23.5915215910775));
#22145=CARTESIAN_POINT('Ctrl Pts',(-1.63737926261779,0.638554747675423,
23.6285659637413));
#22146=CARTESIAN_POINT('Ctrl Pts',(-1.66642057657324,0.0878837734537999,
23.6656103364052));
#22147=CARTESIAN_POINT('Ctrl Pts',(-1.66795453242439,0.0587974530393284,
23.6675670120668));
#22148=CARTESIAN_POINT('Ctrl Pts',(-1.6686516491224,0.0296669993588705,
23.6695236877285));
#22149=CARTESIAN_POINT('Ctrl Pts',(-1.66853019577507,0.000530614451512978,
23.6714803633902));
#22150=CARTESIAN_POINT('Origin',(0.,0.,23.));
#22151=CARTESIAN_POINT('',(-1.66422209409782,0.00118661478516524,24.3714803633902));
#22152=CARTESIAN_POINT('',(-1.66367848409818,-0.000827345116924024,24.1785196366098));
#22153=CARTESIAN_POINT('',(-1.666,2.04026156737949E-16,23.));
#22154=CARTESIAN_POINT('Ctrl Pts',(-1.66367848409818,-0.000827345116924024,
24.1785196366098));
#22155=CARTESIAN_POINT('Ctrl Pts',(-1.66219049440645,0.330217676389022,
24.1564535875851));
#22156=CARTESIAN_POINT('Ctrl Pts',(-1.56660725193993,0.662054420660071,
24.1343875385604));
#22157=CARTESIAN_POINT('Ctrl Pts',(-1.38271566821857,0.93422600678436,24.1123214895358));
#22158=CARTESIAN_POINT('Ctrl Pts',(-1.0739993978296,1.3911463033731,24.0752771168719));
#22159=CARTESIAN_POINT('Ctrl Pts',(-0.516399081127575,1.67990914425084,
24.0382327442081));
#22160=CARTESIAN_POINT('Ctrl Pts',(0.0349164034973534,1.66837097063458,
24.0011883715442));
#22161=CARTESIAN_POINT('Ctrl Pts',(0.586231888122278,1.65683279701833,23.9641439988803));
#22162=CARTESIAN_POINT('Ctrl Pts',(1.13126254067011,1.34499360890808,23.9270996262165));
#22163=CARTESIAN_POINT('Ctrl Pts',(1.42059160843624,0.875557155718521,23.8900552535526));
#22164=CARTESIAN_POINT('Ctrl Pts',(1.70992067620237,0.406120702528958,23.8530108808888));
#22165=CARTESIAN_POINT('Ctrl Pts',(1.7435481591868,-0.220913015739925,23.8159665082249));
#22166=CARTESIAN_POINT('Ctrl Pts',(1.50608545939344,-0.718601029704961,
23.7789221355611));
#22167=CARTESIAN_POINT('Ctrl Pts',(1.26862275960007,-1.21628904367,23.7418777628972));
#22168=CARTESIAN_POINT('Ctrl Pts',(0.760069877028919,-1.58463135333119,
23.7048333902334));
#22169=CARTESIAN_POINT('Ctrl Pts',(0.213150618967734,-1.65506726888155,
23.6677890175695));
#22170=CARTESIAN_POINT('Ctrl Pts',(-0.333768639093451,-1.72550318443192,
23.6307446449057));
#22171=CARTESIAN_POINT('Ctrl Pts',(-0.919054272644665,-1.49803270587146,
23.5937002722418));
#22172=CARTESIAN_POINT('Ctrl Pts',(-1.27486805746385,-1.07675080076484,
23.556655899578));
#22173=CARTESIAN_POINT('Ctrl Pts',(-1.52503614381627,-0.780552922796213,
23.5306104785886));
#22174=CARTESIAN_POINT('Ctrl Pts',(-1.66176906996994,-0.388547954153529,
23.5045650575992));
#22175=CARTESIAN_POINT('Ctrl Pts',(-1.66497222359982,0.00143386426241622,
23.4785196366098));
#22176=CARTESIAN_POINT('Ctrl Pts',(-1.66853019577507,0.000530614451512978,
23.6714803633902));
#22177=CARTESIAN_POINT('Ctrl Pts',(-1.66635225778858,-0.521951810913478,
23.7065680603924));
#22178=CARTESIAN_POINT('Ctrl Pts',(-1.40094886176378,-1.04634152561339,
23.7416557573946));
#22179=CARTESIAN_POINT('Ctrl Pts',(-0.977667790968778,-1.35234861857636,
23.7767434543967));
#22180=CARTESIAN_POINT('Ctrl Pts',(-0.530782327750313,-1.67542028636924,
23.8137878270606));
#22181=CARTESIAN_POINT('Ctrl Pts',(0.0920799623451787,-1.75507387193934,
23.8508321997244));
#22182=CARTESIAN_POINT('Ctrl Pts',(0.605885037559579,-1.55485832696249,
23.8878765723883));
#22183=CARTESIAN_POINT('Ctrl Pts',(1.11969011277398,-1.35464278198564,23.9249209450521));
#22184=CARTESIAN_POINT('Ctrl Pts',(1.52443797310729,-0.874558106461856,
23.961965317716));
#22185=CARTESIAN_POINT('Ctrl Pts',(1.63490803231072,-0.334300495885159,
23.9990096903798));
#22186=CARTESIAN_POINT('Ctrl Pts',(1.74537809151414,0.205957114691539,24.0360540630437));
#22187=CARTESIAN_POINT('Ctrl Pts',(1.56157034958768,0.806387660321145,24.0730984357075));
#22188=CARTESIAN_POINT('Ctrl Pts',(1.167598846538,1.19222230696557,24.1101428083714));
#22189=CARTESIAN_POINT('Ctrl Pts',(0.773627343488314,1.57805695360998,24.1471871810353));
#22190=CARTESIAN_POINT('Ctrl Pts',(0.169492079315405,1.74929570126922,24.1842315536991));
#22191=CARTESIAN_POINT('Ctrl Pts',(-0.368342759829064,1.62757632906868,
24.221275926363));
#22192=CARTESIAN_POINT('Ctrl Pts',(-0.906177598973534,1.50585695686814,
24.2583202990268));
#22193=CARTESIAN_POINT('Ctrl Pts',(-1.37771201308956,1.09117946480783,24.2953646716907));
#22194=CARTESIAN_POINT('Ctrl Pts',(-1.56716257457082,0.573308434028074,
24.3324090443545));
#22195=CARTESIAN_POINT('Ctrl Pts',(-1.63376813250798,0.39123935661342,24.3454328173664));
#22196=CARTESIAN_POINT('Ctrl Pts',(-1.66550726908954,0.196415244238198,
24.3584565903783));
#22197=CARTESIAN_POINT('Ctrl Pts',(-1.66422209409782,0.00118661478516524,
24.3714803633902));
#22198=CARTESIAN_POINT('Origin',(0.,0.,23.));
#22199=CARTESIAN_POINT('',(-1.66424525785499,-0.00119753195345899,25.0714803633902));
#22200=CARTESIAN_POINT('',(-1.66799179081971,-0.000987328612398951,24.8785196366098));
#22201=CARTESIAN_POINT('',(-1.666,2.04026156737949E-16,23.));
#22202=CARTESIAN_POINT('Ctrl Pts',(-1.66799179081971,-0.000987328612398951,
24.8785196366098));
#22203=CARTESIAN_POINT('Ctrl Pts',(-1.66452448203087,0.492811694213693,
24.8453864902349));
#22204=CARTESIAN_POINT('Ctrl Pts',(-1.43140513105353,0.989454702814845,
24.81225334386));
#22205=CARTESIAN_POINT('Ctrl Pts',(-1.04745790195205,1.29904303028329,24.7791201974851));
#22206=CARTESIAN_POINT('Ctrl Pts',(-0.618187343787852,1.64517693635291,
24.7420758248212));
#22207=CARTESIAN_POINT('Ctrl Pts',(-0.000377979727074346,1.75748758204953,
24.7050314521574));
#22208=CARTESIAN_POINT('Ctrl Pts',(0.523248466866253,1.58457940565043,24.6679870794936));
#22209=CARTESIAN_POINT('Ctrl Pts',(1.04687491345958,1.41167122925133,24.6309427068297));
#22210=CARTESIAN_POINT('Ctrl Pts',(1.47631844258546,0.953544230756513,24.5938983341658));
#22211=CARTESIAN_POINT('Ctrl Pts',(1.61505724394959,0.419846340528664,24.556853961502));
#22212=CARTESIAN_POINT('Ctrl Pts',(1.75379604531373,-0.113851549699185,
24.5198095888381));
#22213=CARTESIAN_POINT('Ctrl Pts',(1.60183011891612,-0.72312033166006,24.4827652161743));
#22214=CARTESIAN_POINT('Ctrl Pts',(1.2287020633366,-1.12914662043587,24.4457208435104));
#22215=CARTESIAN_POINT('Ctrl Pts',(0.855574007757078,-1.53517290921169,
24.4086764708466));
#22216=CARTESIAN_POINT('Ctrl Pts',(0.261283822995645,-1.73795670480244,
24.3716320981827));
#22217=CARTESIAN_POINT('Ctrl Pts',(-0.282209606884,-1.6447001515996,24.3345877255189));
#22218=CARTESIAN_POINT('Ctrl Pts',(-0.825703036763652,-1.55144359839676,
24.297543352855));
#22219=CARTESIAN_POINT('Ctrl Pts',(-1.31839971176152,-1.16214669640031,
24.2604989801912));
#22220=CARTESIAN_POINT('Ctrl Pts',(-1.53483193722248,-0.654959369252205,
24.2234546075273));
#22221=CARTESIAN_POINT('Ctrl Pts',(-1.622342986426,-0.449885956330785,24.2084762838881));
#22222=CARTESIAN_POINT('Ctrl Pts',(-1.66468852405365,-0.22553904886167,
24.193497960249));
#22223=CARTESIAN_POINT('Ctrl Pts',(-1.66367848409818,-0.000827345116924024,
24.1785196366098));
#22224=CARTESIAN_POINT('Ctrl Pts',(-1.66422209409782,0.00118661478516524,
24.3714803633902));
#22225=CARTESIAN_POINT('Ctrl Pts',(-1.6618517614814,-0.35888636440512,24.3955009630422));
#22226=CARTESIAN_POINT('Ctrl Pts',(-1.54714313437419,-0.720335383138663,
24.4195215626941));
#22227=CARTESIAN_POINT('Ctrl Pts',(-1.3316535181475,-1.0056739050351,24.4435421623461));
#22228=CARTESIAN_POINT('Ctrl Pts',(-0.999327191396451,-1.4457206438193,
24.4805865350099));
#22229=CARTESIAN_POINT('Ctrl Pts',(-0.427307829047882,-1.7047495518885,
24.5176309076738));
#22230=CARTESIAN_POINT('Ctrl Pts',(0.122637251456149,-1.66422390327097,
24.5546752803376));
#22231=CARTESIAN_POINT('Ctrl Pts',(0.672582331960171,-1.62369825465344,
24.5917196530015));
#22232=CARTESIAN_POINT('Ctrl Pts',(1.20045313061966,-1.28361804934919,24.6287640256653));
#22233=CARTESIAN_POINT('Ctrl Pts',(1.46468558157194,-0.799610682018708,
24.6658083983292));
#22234=CARTESIAN_POINT('Ctrl Pts',(1.72891803252422,-0.315603314688219,
24.702852770993));
#22235=CARTESIAN_POINT('Ctrl Pts',(1.7295121357693,0.31233121466851,24.7398971436569));
#22236=CARTESIAN_POINT('Ctrl Pts',(1.46619601797039,0.796837707786795,24.7769415163208));
#22237=CARTESIAN_POINT('Ctrl Pts',(1.20287990017147,1.28134420090509,24.8139858889846));
#22238=CARTESIAN_POINT('Ctrl Pts',(0.675653561328557,1.62242265778493,24.8510302616485));
#22239=CARTESIAN_POINT('Ctrl Pts',(0.125786149809405,1.66398886419934,24.8880746343123));
#22240=CARTESIAN_POINT('Ctrl Pts',(-0.424081261709735,1.70555507061376,
24.9251190069762));
#22241=CARTESIAN_POINT('Ctrl Pts',(-0.996589745905115,1.44760902656276,
24.96216337964));
#22242=CARTESIAN_POINT('Ctrl Pts',(-1.32974815355174,1.00819191813303,24.9992077523039));
#22243=CARTESIAN_POINT('Ctrl Pts',(-1.54640929346339,0.722428121020488,
25.023298622666));
#22244=CARTESIAN_POINT('Ctrl Pts',(-1.6618439702268,0.35991618045346,25.0473894930281));
#22245=CARTESIAN_POINT('Ctrl Pts',(-1.66424525785499,-0.00119753195345899,
25.0714803633902));
#22246=CARTESIAN_POINT('Origin',(0.,0.,23.));
#22247=CARTESIAN_POINT('',(-1.66854406988197,-0.000512450462931708,25.7714803633902));
#22248=CARTESIAN_POINT('',(-1.66667079046023,0.00145441940323589,25.5785196366098));
#22249=CARTESIAN_POINT('',(-1.666,2.04026156737949E-16,23.));
#22250=CARTESIAN_POINT('Ctrl Pts',(-1.66667079046023,0.00145441940323589,
25.5785196366098));
#22251=CARTESIAN_POINT('Ctrl Pts',(-1.66764896339718,0.108321756637489,
25.5713637655485));
#22252=CARTESIAN_POINT('Ctrl Pts',(-1.65825057352537,0.215017733667649,
25.5642078944873));
#22253=CARTESIAN_POINT('Ctrl Pts',(-1.63785151142752,0.31956732843442,25.557052023426));
#22254=CARTESIAN_POINT('Ctrl Pts',(-1.53225004769563,0.86079761573817,25.5200076507622));
#22255=CARTESIAN_POINT('Ctrl Pts',(-1.13184096675627,1.34450688726362,25.4829632780983));
#22256=CARTESIAN_POINT('Ctrl Pts',(-0.619859344020208,1.54934026105344,
25.4459189054345));
#22257=CARTESIAN_POINT('Ctrl Pts',(-0.107877721284147,1.75417363484326,
25.4088745327706));
#22258=CARTESIAN_POINT('Ctrl Pts',(0.515676443248609,1.68013111089743,25.3718301601067));
#22259=CARTESIAN_POINT('Ctrl Pts',(0.965452492460973,1.36109600531707,25.3347857874429));
#22260=CARTESIAN_POINT('Ctrl Pts',(1.41522854167333,1.04206089973671,25.297741414779));
#22261=CARTESIAN_POINT('Ctrl Pts',(1.69122647556531,0.478033212521821,25.2606970421152));
#22262=CARTESIAN_POINT('Ctrl Pts',(1.66714420800178,-0.0728768867017734,
25.2236526694514));
#22263=CARTESIAN_POINT('Ctrl Pts',(1.64306194043825,-0.623786985925368,
25.1866082967875));
#22264=CARTESIAN_POINT('Ctrl Pts',(1.31889947141923,-1.16157949715767,25.1495639241236));
#22265=CARTESIAN_POINT('Ctrl Pts',(0.842999926222902,-1.44014998360507,
25.1125195514598));
#22266=CARTESIAN_POINT('Ctrl Pts',(0.367100381026566,-1.71872047005247,
25.0754751787959));
#22267=CARTESIAN_POINT('Ctrl Pts',(-0.260536240347081,-1.73806893171496,
25.0384308061321));
#22268=CARTESIAN_POINT('Ctrl Pts',(-0.752691068189035,-1.48934113176189,
25.0013864334682));
#22269=CARTESIAN_POINT('Ctrl Pts',(-1.24484589603098,-1.24061333180882,
24.9643420608044));
#22270=CARTESIAN_POINT('Ctrl Pts',(-1.60151893034123,-0.723809270240203,
24.9272976881405));
#22271=CARTESIAN_POINT('Ctrl Pts',(-1.65948957136256,-0.175428656234587,
24.8902533154767));
#22272=CARTESIAN_POINT('Ctrl Pts',(-1.66561023906039,-0.117529425673589,
24.8863420891877));
#22273=CARTESIAN_POINT('Ctrl Pts',(-1.66840109179986,-0.059278192319831,
24.8824308628988));
#22274=CARTESIAN_POINT('Ctrl Pts',(-1.66799179081971,-0.000987328612398951,
24.8785196366098));
#22275=CARTESIAN_POINT('Ctrl Pts',(-1.66424525785499,-0.00119753195345899,
25.0714803633902));
#22276=CARTESIAN_POINT('Ctrl Pts',(-1.66553641439486,-0.195365996377658,
25.0844338656919));
#22277=CARTESIAN_POINT('Ctrl Pts',(-1.6341480123673,-0.389130213177341,
25.0973873679937));
#22278=CARTESIAN_POINT('Ctrl Pts',(-1.56824460840503,-0.570341953455574,
25.1103408702954));
#22279=CARTESIAN_POINT('Ctrl Pts',(-1.37977432451382,-1.08857054380597,
25.1473852429593));
#22280=CARTESIAN_POINT('Ctrl Pts',(-0.909025425633515,-1.50413955169827,
25.1844296156231));
#22281=CARTESIAN_POINT('Ctrl Pts',(-0.371421872139759,-1.62687642080162,
25.221473988287));
#22282=CARTESIAN_POINT('Ctrl Pts',(0.166181681353993,-1.74961328990496,
25.2585183609509));
#22283=CARTESIAN_POINT('Ctrl Pts',(0.770639889461195,-1.57951802021935,
25.2955627336147));
#22284=CARTESIAN_POINT('Ctrl Pts',(1.16534078053029,-1.19442955459708,25.3326071062786));
#22285=CARTESIAN_POINT('Ctrl Pts',(1.56004167159939,-0.809341088974802,
25.3696514789424));
#22286=CARTESIAN_POINT('Ctrl Pts',(1.74498524563038,-0.209259427415868,
25.4066958516063));
#22287=CARTESIAN_POINT('Ctrl Pts',(1.63553768349278,0.331206252261941,25.4437402242701));
#22288=CARTESIAN_POINT('Ctrl Pts',(1.52609012135517,0.871671931939749,25.480784596934));
#22289=CARTESIAN_POINT('Ctrl Pts',(1.12225142304897,1.35252162973643,25.5178289695978));
#22290=CARTESIAN_POINT('Ctrl Pts',(0.608826124386921,1.55370906090346,25.5548733422617));
#22291=CARTESIAN_POINT('Ctrl Pts',(0.0954008257248699,1.75489649207049,
25.5919177149255));
#22292=CARTESIAN_POINT('Ctrl Pts',(-0.527611073293032,1.67642165660788,
25.6289620875894));
#22293=CARTESIAN_POINT('Ctrl Pts',(-0.975107066920903,1.35419618360633,
25.6660064602532));
#22294=CARTESIAN_POINT('Ctrl Pts',(-1.3998152901679,1.04837934932822,25.7011644279656));
#22295=CARTESIAN_POINT('Ctrl Pts',(-1.66642801081486,0.523004752093186,
25.7363223956779));
#22296=CARTESIAN_POINT('Ctrl Pts',(-1.66854406988197,-0.000512450462931708,
25.7714803633902));
#22297=CARTESIAN_POINT('Origin',(0.,0.,23.));
#22298=CARTESIAN_POINT('',(-1.66575472391166,0.00152194406742107,26.4714803633902));
#22299=CARTESIAN_POINT('',(-1.6632751401947,7.36886941808092E-5,26.2785196366098));
#22300=CARTESIAN_POINT('',(-1.666,2.04026156737949E-16,23.));
#22301=CARTESIAN_POINT('Ctrl Pts',(-1.6632751401947,7.36886941808092E-5,
26.2785196366098));
#22302=CARTESIAN_POINT('Ctrl Pts',(-1.66338307846009,0.273628708276909,
26.2602966681983));
#22303=CARTESIAN_POINT('Ctrl Pts',(-1.59965833684018,0.54713637489195,26.2420736997869));
#22304=CARTESIAN_POINT('Ctrl Pts',(-1.47182530479114,0.786391202256148,
26.2238507313754));
#22305=CARTESIAN_POINT('Ctrl Pts',(-1.21196124910893,1.27275790093975,26.1868063587115));
#22306=CARTESIAN_POINT('Ctrl Pts',(-0.687173720229887,1.61757689837527,
26.1497619860477));
#22307=CARTESIAN_POINT('Ctrl Pts',(-0.137615819036478,1.66305223528393,
26.1127176133838));
#22308=CARTESIAN_POINT('Ctrl Pts',(0.411942082156932,1.70852757219258,26.07567324072));
#22309=CARTESIAN_POINT('Ctrl Pts',(0.986270355664704,1.45465924857437,26.0386288680561));
#22310=CARTESIAN_POINT('Ctrl Pts',(1.32254508083313,1.01762240543881,26.0015844953923));
#22311=CARTESIAN_POINT('Ctrl Pts',(1.65881980600156,0.580585562303244,25.9645401227284));
#22312=CARTESIAN_POINT('Ctrl Pts',(1.75704098283065,-0.0396198003496655,
25.9274957500645));
#22313=CARTESIAN_POINT('Ctrl Pts',(1.57226066784314,-0.559175503069151,
25.8904513774007));
#22314=CARTESIAN_POINT('Ctrl Pts',(1.38748035285563,-1.07873120578864,25.8534070047368));
#22315=CARTESIAN_POINT('Ctrl Pts',(0.919698546051532,-1.4976372485747,25.816362632073));
#22316=CARTESIAN_POINT('Ctrl Pts',(0.382981408073537,-1.62419398224651,
25.7793182594092));
#22317=CARTESIAN_POINT('Ctrl Pts',(-0.153735729904462,-1.75075071591832,
25.7422738867453));
#22318=CARTESIAN_POINT('Ctrl Pts',(-0.759388199056355,-1.58495814047587,
25.7052295140814));
#22319=CARTESIAN_POINT('Ctrl Pts',(-1.15681751037009,-1.20268620121362,
25.6681851414176));
#22320=CARTESIAN_POINT('Ctrl Pts',(-1.47747529869075,-0.894257831459795,
25.638296639815));
#22321=CARTESIAN_POINT('Ctrl Pts',(-1.6625851769628,-0.444906974317528,
25.6084081382124));
#22322=CARTESIAN_POINT('Ctrl Pts',(-1.66667079046023,0.00145441940323589,
25.5785196366098));
#22323=CARTESIAN_POINT('Ctrl Pts',(-1.66854406988197,-0.000512450462931708,
25.7714803633902));
#22324=CARTESIAN_POINT('Ctrl Pts',(-1.66865760728364,-0.0286018284153655,
25.7733667683417));
#22325=CARTESIAN_POINT('Ctrl Pts',(-1.66800969269827,-0.0566858591665887,
25.7752531732933));
#22326=CARTESIAN_POINT('Ctrl Pts',(-1.66658389074195,-0.084730341556093,
25.7771395782448));
#22327=CARTESIAN_POINT('Ctrl Pts',(-1.63858463269728,-0.635455283176455,
25.8141839509086));
#22328=CARTESIAN_POINT('Ctrl Pts',(-1.31060602837012,-1.1709290558767,25.8512283235725));
#22329=CARTESIAN_POINT('Ctrl Pts',(-0.832737541654405,-1.44610832319883,
25.8882726962363));
#22330=CARTESIAN_POINT('Ctrl Pts',(-0.354869054938685,-1.72128759052096,
25.9253170689002));
#22331=CARTESIAN_POINT('Ctrl Pts',(0.272889314165587,-1.73617235246498,
25.9623614415641));
#22332=CARTESIAN_POINT('Ctrl Pts',(0.763262981787752,-1.48395104913065,
25.9994058142279));
#22333=CARTESIAN_POINT('Ctrl Pts',(1.25363664940992,-1.23172974579632,26.0364501868918));
#22334=CARTESIAN_POINT('Ctrl Pts',(1.60662561554998,-0.712402377183643,
26.0734945595556));
#22335=CARTESIAN_POINT('Ctrl Pts',(1.66069518255521,-0.163623367250885,
26.1105389322195));
#22336=CARTESIAN_POINT('Ctrl Pts',(1.71476474956044,0.38515564268187,26.1475833048833));
#22337=CARTESIAN_POINT('Ctrl Pts',(1.46991491743084,0.963386293934705,26.1846276775472));
#22338=CARTESIAN_POINT('Ctrl Pts',(1.03819378793103,1.30645886067622,26.221672050211));
#22339=CARTESIAN_POINT('Ctrl Pts',(0.606472658431218,1.64953142741774,26.2587164228749));
#22340=CARTESIAN_POINT('Ctrl Pts',(-0.01211976843881,1.75744590964794,26.2957607955387));
#22341=CARTESIAN_POINT('Ctrl Pts',(-0.534503424332941,1.58081851723447,
26.3328051682026));
#22342=CARTESIAN_POINT('Ctrl Pts',(-1.05688708022707,1.404191124821,26.3698495408664));
#22343=CARTESIAN_POINT('Ctrl Pts',(-1.4830619651453,0.943021857763867,26.4068939135303));
#22344=CARTESIAN_POINT('Ctrl Pts',(-1.61800206476684,0.408350847098134,
26.4439382861942));
#22345=CARTESIAN_POINT('Ctrl Pts',(-1.65144421691543,0.275843539498134,
26.4531189785928));
#22346=CARTESIAN_POINT('Ctrl Pts',(-1.66699886974927,0.138821790441243,
26.4622996709915));
#22347=CARTESIAN_POINT('Ctrl Pts',(-1.66575472391166,0.00152194406742107,
26.4714803633902));
#22348=CARTESIAN_POINT('Origin',(0.,0.,23.));
#22349=CARTESIAN_POINT('',(-1.66337010699017,-0.000419830789558373,27.1714803633902));
#22350=CARTESIAN_POINT('',(-1.66640033905111,-0.0014929403423002,26.9785196366098));
#22351=CARTESIAN_POINT('',(-1.666,2.04026156737949E-16,23.));
#22352=CARTESIAN_POINT('Ctrl Pts',(-1.66640033905111,-0.0014929403423002,
26.9785196366098));
#22353=CARTESIAN_POINT('Ctrl Pts',(-1.66236155042919,0.436113957710351,
26.9492295708481));
#22354=CARTESIAN_POINT('Ctrl Pts',(-1.48537353306325,0.87661185904339,26.9199395050864));
#22355=CARTESIAN_POINT('Ctrl Pts',(-1.17604733024994,1.18388915163694,26.8906494393248));
#22356=CARTESIAN_POINT('Ctrl Pts',(-0.784829528796659,1.57251561053903,
26.8536050666609));
#22357=CARTESIAN_POINT('Ctrl Pts',(-0.181927270299917,1.74804611280028,
26.816560693997));
#22358=CARTESIAN_POINT('Ctrl Pts',(0.356759509300449,1.63015444211313,26.7795163213332));
#22359=CARTESIAN_POINT('Ctrl Pts',(0.895446288900814,1.51226277142598,26.7424719486693));
#22360=CARTESIAN_POINT('Ctrl Pts',(1.36991758960481,1.10094892779044,26.7054275760055));
#22361=CARTESIAN_POINT('Ctrl Pts',(1.56304600538008,0.584438222746841,26.6683832033416));
#22362=CARTESIAN_POINT('Ctrl Pts',(1.75617442115535,0.0679275177032342,
26.6313388306778));
#22363=CARTESIAN_POINT('Ctrl Pts',(1.6679599520019,-0.553780048748435,26.5942944580139));
#22364=CARTESIAN_POINT('Ctrl Pts',(1.33877127573794,-0.996178860214455,
26.55725008535));
#22365=CARTESIAN_POINT('Ctrl Pts',(1.00958259947398,-1.43857767168047,26.5202057126862));
#22366=CARTESIAN_POINT('Ctrl Pts',(0.439419716099504,-1.70166772816084,
26.4831613400223));
#22367=CARTESIAN_POINT('Ctrl Pts',(-0.110799618615914,-1.66505384167596,
26.4461169673585));
#22368=CARTESIAN_POINT('Ctrl Pts',(-0.661018953331337,-1.62843995519108,
26.4090725946946));
#22369=CARTESIAN_POINT('Ctrl Pts',(-1.1912947393877,-1.29212212574094,26.3720282220308));
#22370=CARTESIAN_POINT('Ctrl Pts',(-1.4589623411732,-0.810006011050031,
26.3349838493669));
#22371=CARTESIAN_POINT('Ctrl Pts',(-1.59495816931649,-0.565053764901262,
26.3161624451146));
#22372=CARTESIAN_POINT('Ctrl Pts',(-1.66316365727483,-0.282464781031254,
26.2973410408622));
#22373=CARTESIAN_POINT('Ctrl Pts',(-1.6632751401947,7.36886941808092E-5,
26.2785196366098));
#22374=CARTESIAN_POINT('Ctrl Pts',(-1.66575472391166,0.00152194406742107,
26.4714803633902));
#22375=CARTESIAN_POINT('Ctrl Pts',(-1.66197870350743,-0.415187259735411,
26.4993440436554));
#22376=CARTESIAN_POINT('Ctrl Pts',(-1.50346207181111,-0.834458131765972,
26.5272077239205));
#22377=CARTESIAN_POINT('Ctrl Pts',(-1.22064153164464,-1.13785559215971,
26.5550714041857));
#22378=CARTESIAN_POINT('Ctrl Pts',(-0.844635584576064,-1.54121826647749,
26.5921157768495));
#22379=CARTESIAN_POINT('Ctrl Pts',(-0.24891837611407,-1.73977086083872,
26.6291601495134));
#22380=CARTESIAN_POINT('Ctrl Pts',(0.29389817533508,-1.64265180536657,26.6662045221773));
#22381=CARTESIAN_POINT('Ctrl Pts',(0.836714726784226,-1.54553274989443,
26.7032488948411));
#22382=CARTESIAN_POINT('Ctrl Pts',(1.32663062122053,-1.15274204458891,26.740293267505));
#22383=CARTESIAN_POINT('Ctrl Pts',(1.53945070430983,-0.64402843705345,26.7773376401688));
#22384=CARTESIAN_POINT('Ctrl Pts',(1.75227078739912,-0.135314829517993,
26.8143820128327));
#22385=CARTESIAN_POINT('Ctrl Pts',(1.68799505914141,0.489321680247402,26.8514263854965));
#22386=CARTESIAN_POINT('Ctrl Pts',(1.37603735693171,0.944035114977717,26.8884707581604));
#22387=CARTESIAN_POINT('Ctrl Pts',(1.06407965472201,1.39874854970803,26.9255151308242));
#22388=CARTESIAN_POINT('Ctrl Pts',(0.504439978560328,1.68353890940327,26.9625595034881));
#22389=CARTESIAN_POINT('Ctrl Pts',(-0.0467795406218917,1.66808055482026,
26.9996038761519));
#22390=CARTESIAN_POINT('Ctrl Pts',(-0.597999059804111,1.65262220023726,
27.0366482488158));
#22391=CARTESIAN_POINT('Ctrl Pts',(-1.14079842200687,1.33691513137601,27.0736926214796));
#22392=CARTESIAN_POINT('Ctrl Pts',(-1.42678195981814,0.865433050682779,
27.1107369941435));
#22393=CARTESIAN_POINT('Ctrl Pts',(-1.58309543279269,0.607729400876687,
27.1309847838924));
#22394=CARTESIAN_POINT('Ctrl Pts',(-1.66268467615298,0.303487661744212,
27.1512325736413));
#22395=CARTESIAN_POINT('Ctrl Pts',(-1.66337010699017,-0.000419830789558373,
27.1714803633902));
#22396=CARTESIAN_POINT('Origin',(0.,0.,23.));
#22397=CARTESIAN_POINT('',(-1.66729377121886,-0.00130306451899955,27.8714803633902));
#22398=CARTESIAN_POINT('',(-1.66818493320164,0.000858898907110364,27.6785196366098));
#22399=CARTESIAN_POINT('',(-1.666,2.04026156737949E-16,23.));
#22400=CARTESIAN_POINT('Ctrl Pts',(-1.66818493320164,0.000858898907110364,
27.6785196366098));
#22401=CARTESIAN_POINT('Ctrl Pts',(-1.66849498077994,0.0502159495743163,
27.6752068461618));
#22402=CARTESIAN_POINT('Ctrl Pts',(-1.66649429024572,0.0995475114464373,
27.6718940557137));
#22403=CARTESIAN_POINT('Ctrl Pts',(-1.66210102607721,0.148665069498833,
27.6685812652656));
#22404=CARTESIAN_POINT('Ctrl Pts',(-1.61297455169828,0.697908721749858,
27.6315368926018));
#22405=CARTESIAN_POINT('Ctrl Pts',(-1.26467543919903,1.22039286850551,27.5944925199379));
#22406=CARTESIAN_POINT('Ctrl Pts',(-0.776592464269594,1.47701887638357,
27.5574481472741));
#22407=CARTESIAN_POINT('Ctrl Pts',(-0.288509489340157,1.73364488426163,
27.5204037746102));
#22408=CARTESIAN_POINT('Ctrl Pts',(0.339357348019464,1.72441275326209,27.4833594019464));
#22409=CARTESIAN_POINT('Ctrl Pts',(0.819683955401358,1.45354708297435,27.4463150292825));
#22410=CARTESIAN_POINT('Ctrl Pts',(1.30001056278325,1.18268141268661,27.4092706566187));
#22411=CARTESIAN_POINT('Ctrl Pts',(1.63279694018742,0.650182203110672,27.3722262839548));
#22412=CARTESIAN_POINT('Ctrl Pts',(1.66575342521178,0.0997316787937973,
27.335181911291));
#22413=CARTESIAN_POINT('Ctrl Pts',(1.69870991023614,-0.450718845523074,
27.2981375386271));
#22414=CARTESIAN_POINT('Ctrl Pts',(1.4318365028807,-1.01912068458088,27.2610931659632));
#22415=CARTESIAN_POINT('Ctrl Pts',(0.987259761184316,-1.34536202632351,
27.2240487932994));
#22416=CARTESIAN_POINT('Ctrl Pts',(0.542683019487933,-1.67160336806614,
27.1870044206355));
#22417=CARTESIAN_POINT('Ctrl Pts',(-0.0795970565493923,-1.75568421249359,
27.1499600479717));
#22418=CARTESIAN_POINT('Ctrl Pts',(-0.594812875890746,-1.55912748161231,
27.1129156753079));
#22419=CARTESIAN_POINT('Ctrl Pts',(-1.1100286952321,-1.36257075073103,27.075871302644));
#22420=CARTESIAN_POINT('Ctrl Pts',(-1.51818025787748,-0.885376444541015,
27.0388269299801));
#22421=CARTESIAN_POINT('Ctrl Pts',(-1.63248936699526,-0.345918083674546,
27.0017825573163));
#22422=CARTESIAN_POINT('Ctrl Pts',(-1.65641710149505,-0.232996055569109,
26.9940282504141));
#22423=CARTESIAN_POINT('Ctrl Pts',(-1.66746957551995,-0.117345810650349,
26.986273943512));
#22424=CARTESIAN_POINT('Ctrl Pts',(-1.66640033905111,-0.0014929403423002,
26.9785196366098));
#22425=CARTESIAN_POINT('Ctrl Pts',(-1.66337010699017,-0.000419830789558373,
27.1714803633902));
#22426=CARTESIAN_POINT('Ctrl Pts',(-1.66393870712045,-0.252526725424533,
27.1882769463052));
#22427=CARTESIAN_POINT('Ctrl Pts',(-1.61020920893848,-0.504403606399881,
27.2050735292201));
#22428=CARTESIAN_POINT('Ctrl Pts',(-1.5009373747887,-0.729292911466197,
27.2218701121351));
#22429=CARTESIAN_POINT('Ctrl Pts',(-1.2599415385282,-1.22527970039674,27.2589144847989));
#22430=CARTESIAN_POINT('Ctrl Pts',(-0.748782152587401,-1.58999618573263,
27.2959588574628));
#22431=CARTESIAN_POINT('Ctrl Pts',(-0.201375822283328,-1.65654116769859,
27.3330032301266));
#22432=CARTESIAN_POINT('Ctrl Pts',(0.346030508020746,-1.72308614966455,
27.3700476027905));
#22433=CARTESIAN_POINT('Ctrl Pts',(0.929683782688092,-1.49145962826058,
27.4070919754543));
#22434=CARTESIAN_POINT('Ctrl Pts',(1.28249279779562,-1.06765799378737,27.4441363481182));
#22435=CARTESIAN_POINT('Ctrl Pts',(1.63530181290315,-0.643856359314169,
27.481180720782));
#22436=CARTESIAN_POINT('Ctrl Pts',(1.75726656845087,-0.0278796117717245,
27.5182250934459));
#22437=CARTESIAN_POINT('Ctrl Pts',(1.59257355216309,0.498388274239166,27.5552694661097));
#22438=CARTESIAN_POINT('Ctrl Pts',(1.42788053587531,1.02465616025006,27.5923138387736));
#22439=CARTESIAN_POINT('Ctrl Pts',(0.97652974775204,1.46121518472939,27.6293582114374));
#22440=CARTESIAN_POINT('Ctrl Pts',(0.445068267638841,1.60828906290049,27.6664025841013));
#22441=CARTESIAN_POINT('Ctrl Pts',(-0.0863932124743599,1.75536294107158,
27.7034469567652));
#22442=CARTESIAN_POINT('Ctrl Pts',(-0.69796538457749,1.61295167293442,27.740491329429));
#22443=CARTESIAN_POINT('Ctrl Pts',(-1.10978093456905,1.24622215767095,27.7775357020928));
#22444=CARTESIAN_POINT('Ctrl Pts',(-1.45790283612392,0.93621303778115,27.808850589192));
#22445=CARTESIAN_POINT('Ctrl Pts',(-1.66328056200809,0.465908239402866,
27.8401654762911));
#22446=CARTESIAN_POINT('Ctrl Pts',(-1.66729377121886,-0.00130306451899955,
27.8714803633902));
#22447=CARTESIAN_POINT('Origin',(0.,0.,23.));
#22448=CARTESIAN_POINT('',(-1.66745735078673,0.00120170187390745,28.5714803633902));
#22449=CARTESIAN_POINT('',(-1.6638200260918,0.000942871389988137,28.3785196366098));
#22450=CARTESIAN_POINT('',(-1.666,2.04026156737949E-16,23.));
#22451=CARTESIAN_POINT('',(1.26907087985238,1.07935865304851,29.));
#22452=CARTESIAN_POINT('Ctrl Pts',(-1.66745735078673,0.00120170187390745,
28.5714803633902));
#22453=CARTESIAN_POINT('Ctrl Pts',(-1.66350963374581,-0.471613114236158,
28.6031871242686));
#22454=CARTESIAN_POINT('Ctrl Pts',(-1.45232521651817,-0.94739347524418,
28.6348938851469));
#22455=CARTESIAN_POINT('Ctrl Pts',(-1.09656156402175,-1.25768579906275,
28.6666006460253));
#22456=CARTESIAN_POINT('Ctrl Pts',(-0.680907584926055,-1.62021366882408,
28.7036450186892));
#22457=CARTESIAN_POINT('Ctrl Pts',(-0.0678992765999901,-1.75684616353755,
28.740689391353));
#22458=CARTESIAN_POINT('Ctrl Pts',(0.462005451356146,-1.60382582725002,
28.7777337640169));
#22459=CARTESIAN_POINT('Ctrl Pts',(0.991910179312282,-1.45080549096249,
28.8147781366808));
#22460=CARTESIAN_POINT('Ctrl Pts',(1.43871132689849,-1.00813232367397,28.8518225093446));
#22461=CARTESIAN_POINT('Ctrl Pts',(1.59772575664243,-0.481085822244155,
28.8888668820085));
#22462=CARTESIAN_POINT('Ctrl Pts',(1.75674018638636,0.0459606791856584,
28.9259112546723));
#22463=CARTESIAN_POINT('Ctrl Pts',(1.62796789828802,0.657380514756762,28.9629556273361));
#22464=CARTESIAN_POINT('Ctrl Pts',(1.26907087985237,1.07935865304853,29.));
#22465=CARTESIAN_POINT('',(-1.27144765946785,1.08124504477636,29.));
#22466=CARTESIAN_POINT('Origin',(0.,0.,29.));
#22467=CARTESIAN_POINT('Ctrl Pts',(-1.27144834193525,1.08124558643403,29.));
#22468=CARTESIAN_POINT('Ctrl Pts',(-0.920624410300644,1.49274880387387,
28.9636818543909));
#22469=CARTESIAN_POINT('Ctrl Pts',(-0.350778053489151,1.71868133567313,
28.9273637087819));
#22470=CARTESIAN_POINT('Ctrl Pts',(0.186547721698795,1.65813753251397,28.8910455631728));
#22471=CARTESIAN_POINT('Ctrl Pts',(0.734618002384743,1.59638307977135,28.8540011905089));
#22472=CARTESIAN_POINT('Ctrl Pts',(1.24885411811842,1.23658083427687,28.8169568178451));
#22473=CARTESIAN_POINT('Ctrl Pts',(1.49426097077748,0.742855457794705,28.7799124451812));
#22474=CARTESIAN_POINT('Ctrl Pts',(1.73966782343655,0.249130081312535,28.7428680725174));
#22475=CARTESIAN_POINT('Ctrl Pts',(1.71624541302099,-0.378518426157325,
28.7058236998535));
#22476=CARTESIAN_POINT('Ctrl Pts',(1.43454159545344,-0.852593208110846,
28.6687793271897));
#22477=CARTESIAN_POINT('Ctrl Pts',(1.1528377778859,-1.32666799006437,28.6317349545258));
#22478=CARTESIAN_POINT('Ctrl Pts',(0.612852553166363,-1.64716904650155,
28.594690581862));
#22479=CARTESIAN_POINT('Ctrl Pts',(0.0617825081308379,-1.66757033753488,
28.5576462091981));
#22480=CARTESIAN_POINT('Ctrl Pts',(-0.489287536904685,-1.68797162856822,
28.5206018365343));
#22481=CARTESIAN_POINT('Ctrl Pts',(-1.0514424022562,-1.4082731541977,28.4835574638704));
#22482=CARTESIAN_POINT('Ctrl Pts',(-1.36747510148739,-0.956396832767403,
28.4465130912066));
#22483=CARTESIAN_POINT('Ctrl Pts',(-1.56083020008092,-0.679929901039163,
28.423848606341));
#22484=CARTESIAN_POINT('Ctrl Pts',(-1.66205596190706,-0.339012736706109,
28.4011841214754));
#22485=CARTESIAN_POINT('Ctrl Pts',(-1.6638200260918,0.000942871389988137,
28.3785196366098));
#22486=CARTESIAN_POINT('Origin',(0.,0.,30.5459252805377));
#22487=CARTESIAN_POINT('',(-2.05539098592872,0.00181257412559116,18.3540747194623));
#22488=CARTESIAN_POINT('',(-2.05290622350845,-0.00151880093680796,18.2959252805377));
#22489=CARTESIAN_POINT('',(-2.05475,1.58232769237955E-13,30.5459252805377));
#22490=CARTESIAN_POINT('',(1.81742788875943,0.958620587959298,18.));
#22491=CARTESIAN_POINT('Ctrl Pts',(-2.05290622350845,-0.00151880093680801,
18.2959252805377));
#22492=CARTESIAN_POINT('Ctrl Pts',(-2.04995766327688,0.45238457131471,18.2713722656862));
#22493=CARTESIAN_POINT('Ctrl Pts',(-1.67844748626583,1.5958979401344,18.2097748781708));
#22494=CARTESIAN_POINT('Ctrl Pts',(0.216442804381921,2.41814053114287,18.1111331179916));
#22495=CARTESIAN_POINT('Ctrl Pts',(1.4986774253635,1.56293264739877,18.0370443726639));
#22496=CARTESIAN_POINT('Ctrl Pts',(1.81742788875943,0.958620587959298,18.));
#22497=CARTESIAN_POINT('',(2.0571089891529,-0.0753984945660209,18.));
#22498=CARTESIAN_POINT('Origin',(0.,0.,18.));
#22499=CARTESIAN_POINT('Ctrl Pts',(-2.05539098592872,0.001812574125591,
18.3540747194623));
#22500=CARTESIAN_POINT('Ctrl Pts',(-2.05668615726959,0.142173868935286,
18.3464567039116));
#22501=CARTESIAN_POINT('Ctrl Pts',(-1.97955796804357,0.963669298063719,
18.3017943156971));
#22502=CARTESIAN_POINT('Ctrl Pts',(-0.873549834886296,2.26598780907704,
18.2200875548188));
#22503=CARTESIAN_POINT('Ctrl Pts',(1.41373496756836,1.96497190368407,18.109680663882));
#22504=CARTESIAN_POINT('Ctrl Pts',(2.08071254605835,0.591116081556763,18.0363181456091));
#22505=CARTESIAN_POINT('Ctrl Pts',(2.0571100610898,-0.0753985702550394,
18.));
#22506=CARTESIAN_POINT('Origin',(0.,0.,30.5459252805377));
#22507=CARTESIAN_POINT('',(-2.05138759503762,-4.97339178941181E-5,19.0540747194623));
#22508=CARTESIAN_POINT('',(-2.05798293875546,-0.000483242835675936,18.9959252805377));
#22509=CARTESIAN_POINT('',(-2.05475,1.58232769237955E-13,30.5459252805377));
#22510=CARTESIAN_POINT('Ctrl Pts',(-2.05798293875546,-0.000483242835675884,
18.9959252805377));
#22511=CARTESIAN_POINT('Ctrl Pts',(-2.05591526442115,0.653598076368698,
18.9603051683359));
#22512=CARTESIAN_POINT('Ctrl Pts',(-1.36492080142796,1.99168784117887,18.8876406834704));
#22513=CARTESIAN_POINT('Ctrl Pts',(0.91417845046059,2.24995443991895,18.7779318259409));
#22514=CARTESIAN_POINT('Ctrl Pts',(2.38596583103409,0.452399485900713,18.6667987079494));
#22515=CARTESIAN_POINT('Ctrl Pts',(1.67442227650725,-1.75934857315356,18.5556655899578));
#22516=CARTESIAN_POINT('Ctrl Pts',(-0.570385735669315,-2.36060373212415,
18.4445324719663));
#22517=CARTESIAN_POINT('Ctrl Pts',(-1.91138556361506,-1.14623593643521,
18.3579523688262));
#22518=CARTESIAN_POINT('Ctrl Pts',(-2.05440630490808,-0.232442354288971,
18.30841663835));
#22519=CARTESIAN_POINT('Ctrl Pts',(-2.05290622350845,-0.00151880093680801,
18.2959252805377));
#22520=CARTESIAN_POINT('Ctrl Pts',(-2.05138759503762,-4.97339178940834E-5,
19.0540747194623));
#22521=CARTESIAN_POINT('Ctrl Pts',(-2.05131375814071,0.34589479280389,19.0353896065614));
#22522=CARTESIAN_POINT('Ctrl Pts',(-1.80422891290684,1.37779527947084,18.9796601209967));
#22523=CARTESIAN_POINT('Ctrl Pts',(-0.170134977547301,2.42261514214274,
18.8868862627681));
#22524=CARTESIAN_POINT('Ctrl Pts',(1.9430184348445,1.45691614743391,18.7757531447766));
#22525=CARTESIAN_POINT('Ctrl Pts',(2.27790227156009,-0.842194003777161,
18.664620026785));
#22526=CARTESIAN_POINT('Ctrl Pts',(0.52784999826971,-2.37052551568832,18.5534869087934));
#22527=CARTESIAN_POINT('Ctrl Pts',(-1.55203386772556,-1.77316213953964,
18.4499718063526));
#22528=CARTESIAN_POINT('Ctrl Pts',(-2.05038808535102,-0.540365576925945,
18.3835010765755));
#22529=CARTESIAN_POINT('Ctrl Pts',(-2.05539098592872,0.001812574125591,
18.3540747194623));
#22530=CARTESIAN_POINT('Origin',(0.,0.,30.5459252805377));
#22531=CARTESIAN_POINT('',(-2.05550167136418,-0.00180630479153662,19.7540747194623));
#22532=CARTESIAN_POINT('',(-2.05419418048317,0.00186544829068187,19.6959252805377));
#22533=CARTESIAN_POINT('',(-2.05475,1.58232769237955E-13,30.5459252805377));
#22534=CARTESIAN_POINT('Ctrl Pts',(-2.05419418048317,0.00186544829068198,
19.6959252805377));
#22535=CARTESIAN_POINT('Ctrl Pts',(-2.05577927155616,0.179783416190269,
19.6862824436496));
#22536=CARTESIAN_POINT('Ctrl Pts',(-1.95316269205233,1.03939956340346,19.6395952340976));
#22537=CARTESIAN_POINT('Ctrl Pts',(-0.74919538183736,2.31013209082318,19.5558636518818));
#22538=CARTESIAN_POINT('Ctrl Pts',(1.53447086719707,1.88239297517548,19.4447305338903));
#22539=CARTESIAN_POINT('Ctrl Pts',(2.41372487585493,-0.268184847585669,
19.3335974158987));
#22540=CARTESIAN_POINT('Ctrl Pts',(1.08385077038562,-2.17331209936668,19.2224642979071));
#22541=CARTESIAN_POINT('Ctrl Pts',(-1.23802140067364,-2.08933327590159,
19.1113311799156));
#22542=CARTESIAN_POINT('Ctrl Pts',(-2.04576099362511,-0.732944466062138,
19.0358181741258));
#22543=CARTESIAN_POINT('Ctrl Pts',(-2.05806561414924,-0.0266365058203424,
18.9973495409998));
#22544=CARTESIAN_POINT('Ctrl Pts',(-2.05798293875546,-0.000483242835675884,
18.9959252805377));
#22545=CARTESIAN_POINT('Ctrl Pts',(-2.05550167136418,-0.00180630479153664,
19.7540747194623));
#22546=CARTESIAN_POINT('Ctrl Pts',(-2.05047133330275,0.546252139932218,
19.7243225092112));
#22547=CARTESIAN_POINT('Ctrl Pts',(-1.54308293551855,1.7849188256759,19.6575259262963));
#22548=CARTESIAN_POINT('Ctrl Pts',(0.548689842456826,2.36578558927548,19.5536849707175));
#22549=CARTESIAN_POINT('Ctrl Pts',(2.28517284872419,0.82218308608128,19.4425518527259));
#22550=CARTESIAN_POINT('Ctrl Pts',(1.93017685695003,-1.47391342438527,19.3314187347344));
#22551=CARTESIAN_POINT('Ctrl Pts',(-0.191395150412758,-2.42102695967158,
19.2202856167428));
#22552=CARTESIAN_POINT('Ctrl Pts',(-1.81053783300646,-1.36563128814009,
19.1278376116521));
#22553=CARTESIAN_POINT('Ctrl Pts',(-2.05146014427923,-0.339961270088832,
19.0724339792253));
#22554=CARTESIAN_POINT('Ctrl Pts',(-2.05138759503762,-4.97339178940834E-5,
19.0540747194623));
#22555=CARTESIAN_POINT('Origin',(0.,0.,30.5459252805377));
#22556=CARTESIAN_POINT('',(-2.05726314523298,0.00118285322517675,20.4540747194623));
#22557=CARTESIAN_POINT('',(-2.05157916456917,-0.000651383278007832,20.3959252805377));
#22558=CARTESIAN_POINT('',(-2.05475,1.58232769237955E-13,30.5459252805377));
#22559=CARTESIAN_POINT('Ctrl Pts',(-2.05157916456917,-0.000651383278007581,
20.3959252805377));
#22560=CARTESIAN_POINT('Ctrl Pts',(-2.05048915160027,0.382692054795739,
20.3752153462994));
#22561=CARTESIAN_POINT('Ctrl Pts',(-1.76331355358747,1.45324785939933,20.3174610393972));
#22562=CARTESIAN_POINT('Ctrl Pts',(-0.037864870345937,2.42828507097424,
20.2226623598312));
#22563=CARTESIAN_POINT('Ctrl Pts',(2.01954547577021,1.34886554398611,20.1115292418396));
#22564=CARTESIAN_POINT('Ctrl Pts',(2.22858823263633,-0.965088791301547,
20.0003961238481));
#22565=CARTESIAN_POINT('Ctrl Pts',(0.397939478909703,-2.39575593384446,
19.8892630058565));
#22566=CARTESIAN_POINT('Ctrl Pts',(-1.60647516920198,-1.69985232818512,
19.787772724753));
#22567=CARTESIAN_POINT('Ctrl Pts',(-2.04968991164107,-0.503714560904521,
19.7233268163134));
#22568=CARTESIAN_POINT('Ctrl Pts',(-2.05419418048317,0.00186544829068198,
19.6959252805377));
#22569=CARTESIAN_POINT('Ctrl Pts',(-2.05726314523298,0.00118285322517685,
20.4540747194623));
#22570=CARTESIAN_POINT('Ctrl Pts',(-2.05773933212956,0.0705652968257603,
20.4502997845249));
#22571=CARTESIAN_POINT('Ctrl Pts',(-2.02307416841907,0.820333420006341,
20.4094804769236));
#22572=CARTESIAN_POINT('Ctrl Pts',(-1.10336950687639,2.16346419607446,20.3316167966584));
#22573=CARTESIAN_POINT('Ctrl Pts',(1.21915193180051,2.10039762278245,20.2204836786668));
#22574=CARTESIAN_POINT('Ctrl Pts',(2.42585752542742,0.114964471039976,20.1093505606753));
#22575=CARTESIAN_POINT('Ctrl Pts',(1.41232285348001,-1.97568868333651,19.9982174426837));
#22576=CARTESIAN_POINT('Ctrl Pts',(-0.893825325748239,-2.2581138043306,
19.8870843246922));
#22577=CARTESIAN_POINT('Ctrl Pts',(-1.98352412167925,-0.95150867536627,
19.8057034169517));
#22578=CARTESIAN_POINT('Ctrl Pts',(-2.05673458958522,-0.136133507943197,
19.7613668818751));
#22579=CARTESIAN_POINT('Ctrl Pts',(-2.05550167136418,-0.00180630479153664,
19.7540747194623));
#22580=CARTESIAN_POINT('Origin',(0.,0.,30.5459252805377));
#22581=CARTESIAN_POINT('',(-2.0519251869176,0.00105510962586416,21.1540747194623));
#22582=CARTESIAN_POINT('',(-2.0565803487625,-0.00152072744175304,21.0959252805377));
#22583=CARTESIAN_POINT('',(-2.05475,1.58232769237955E-13,30.5459252805377));
#22584=CARTESIAN_POINT('Ctrl Pts',(-2.0565803487625,-0.00152072744175287,
21.0959252805377));
#22585=CARTESIAN_POINT('Ctrl Pts',(-2.0517372846152,0.583041769572967,21.0641482489491));
#22586=CARTESIAN_POINT('Ctrl Pts',(-1.48486127333146,1.8572733659222,20.9953268446968));
#22587=CARTESIAN_POINT('Ctrl Pts',(0.676803113364313,2.33236782238435,20.8894610677805));
#22588=CARTESIAN_POINT('Ctrl Pts',(2.3265840468287,0.696425723269271,20.778327949789));
#22589=CARTESIAN_POINT('Ctrl Pts',(1.84698368557056,-1.57691260826926,20.6671948317974));
#22590=CARTESIAN_POINT('Ctrl Pts',(-0.323048838197336,-2.40699845512473,
20.5560617138059));
#22591=CARTESIAN_POINT('Ctrl Pts',(-1.84812165816893,-1.28994678035528,
20.4656385300526));
#22592=CARTESIAN_POINT('Ctrl Pts',(-2.0524388848135,-0.303003853981133,
20.4122597189632));
#22593=CARTESIAN_POINT('Ctrl Pts',(-2.05157916456917,-0.000651383278007581,
20.3959252805377));
#22594=CARTESIAN_POINT('Ctrl Pts',(-2.0519251869176,0.00105510962586441,
21.1540747194623));
#22595=CARTESIAN_POINT('Ctrl Pts',(-2.05320297921829,0.275667101474611,
21.1392326871747));
#22596=CARTESIAN_POINT('Ctrl Pts',(-1.87404526463701,1.23408694721642,21.0873462822232));
#22597=CARTESIAN_POINT('Ctrl Pts',(-0.419493009128206,2.39207592060309,
20.9984155046077));
#22598=CARTESIAN_POINT('Ctrl Pts',(1.7821373527842,1.64984485657254,20.8872823866162));
#22599=CARTESIAN_POINT('Ctrl Pts',(2.35268546495377,-0.602389157518069,
20.7761492686246));
#22600=CARTESIAN_POINT('Ctrl Pts',(0.769963239246222,-2.30329290471873,
20.6650161506331));
#22601=CARTESIAN_POINT('Ctrl Pts',(-1.43976118523263,-1.90996263191677,
20.557657967579));
#22602=CARTESIAN_POINT('Ctrl Pts',(-2.05306639202681,-0.6103018279468,20.4873441571887));
#22603=CARTESIAN_POINT('Ctrl Pts',(-2.05726314523298,0.00118285322517685,
20.4540747194623));
#22604=CARTESIAN_POINT('Origin',(0.,0.,30.5459252805377));
#22605=CARTESIAN_POINT('',(-2.05341424816682,-0.00175368872599717,21.8540747194623));
#22606=CARTESIAN_POINT('',(-2.05630909038221,0.00161611837171143,21.7959252805377));
#22607=CARTESIAN_POINT('',(-2.05475,1.58232769237955E-13,30.5459252805377));
#22608=CARTESIAN_POINT('Ctrl Pts',(-2.05630909038221,0.00161611837171153,
21.7959252805377));
#22609=CARTESIAN_POINT('Ctrl Pts',(-2.05723022072092,0.108343634502101,
21.7901255242628));
#22610=CARTESIAN_POINT('Ctrl Pts',(-2.00114645477151,0.895793945750412,
21.747281395324));
#22611=CARTESIAN_POINT('Ctrl Pts',(-0.983827005302519,2.22037981812055,
21.6673928937214));
#22612=CARTESIAN_POINT('Ctrl Pts',(1.33180612413638,2.03083592660637,21.5562597757299));
#22613=CARTESIAN_POINT('Ctrl Pts',(2.42851786940399,-0.0174089378669135,
21.4451266577383));
#22614=CARTESIAN_POINT('Ctrl Pts',(1.30255447502931,-2.04972045718415,21.3339935397468));
#22615=CARTESIAN_POINT('Ctrl Pts',(-1.01555804287549,-2.20604713789681,
21.2228604217552));
#22616=CARTESIAN_POINT('Ctrl Pts',(-2.00713056245277,-0.875936710560245,
21.1435043353522));
#22617=CARTESIAN_POINT('Ctrl Pts',(-2.05738313207606,-0.0984174449039837,
21.101192621613));
#22618=CARTESIAN_POINT('Ctrl Pts',(-2.0565803487625,-0.00152072744175287,
21.0959252805377));
#22619=CARTESIAN_POINT('Ctrl Pts',(-2.05341424816682,-0.0017536887259971,
21.8540747194623));
#22620=CARTESIAN_POINT('Ctrl Pts',(-2.04952656050121,0.476751074253768,
21.8281655898244));
#22621=CARTESIAN_POINT('Ctrl Pts',(-1.64443235649635,1.64534626353278,21.7652120875227));
#22622=CARTESIAN_POINT('Ctrl Pts',(0.301364750346359,2.40980930405301,21.6652142125571));
#22623=CARTESIAN_POINT('Ctrl Pts',(2.18801481710634,1.05384664671037,21.5540810945656));
#22624=CARTESIAN_POINT('Ctrl Pts',(2.07210760382199,-1.2666379407027,21.442947976574));
#22625=CARTESIAN_POINT('Ctrl Pts',(0.0597259541680415,-2.42784563039867,
21.3318148585825));
#22626=CARTESIAN_POINT('Ctrl Pts',(-1.73126155251785,-1.50867220106731,
21.2355237728785));
#22627=CARTESIAN_POINT('Ctrl Pts',(-2.05001372499377,-0.409739638440497,
21.1762770598385));
#22628=CARTESIAN_POINT('Ctrl Pts',(-2.0519251869176,0.00105510962586441,
21.1540747194623));
#22629=CARTESIAN_POINT('Origin',(0.,0.,30.5459252805377));
#22630=CARTESIAN_POINT('',(-2.05812459253004,-2.33768028169005E-5,22.5540747194623));
#22631=CARTESIAN_POINT('',(-2.05149685129519,0.000497173714744954,22.4959252805377));
#22632=CARTESIAN_POINT('',(-2.05475,1.58232769237955E-13,30.5459252805377));
#22633=CARTESIAN_POINT('Ctrl Pts',(-2.05149685129519,0.000497173714744739,
22.4959252805377));
#22634=CARTESIAN_POINT('Ctrl Pts',(-2.05217289056284,0.312735992683416,
22.4790584269126));
#22635=CARTESIAN_POINT('Ctrl Pts',(-1.83851165054927,1.30986170311779,22.4251472006236));
#22636=CARTESIAN_POINT('Ctrl Pts',(-0.288508063209722,2.41138242727093,
22.3341916016708));
#22637=CARTESIAN_POINT('Ctrl Pts',(1.86940104446612,1.5502715400977,22.2230584836792));
#22638=CARTESIAN_POINT('Ctrl Pts',(2.31636073733878,-0.729708878666279,
22.1119253656877));
#22639=CARTESIAN_POINT('Ctrl Pts',(0.643295912328174,-2.34183101061307,
22.0007922476961));
#22640=CARTESIAN_POINT('Ctrl Pts',(-1.50049922779959,-1.83833993148199,
21.8954588859795));
#22641=CARTESIAN_POINT('Ctrl Pts',(-2.05134675011945,-0.573349473558514,
21.8271698969266));
#22642=CARTESIAN_POINT('Ctrl Pts',(-2.05630909038221,0.00161611837171153,
21.7959252805377));
#22643=CARTESIAN_POINT('Ctrl Pts',(-2.05812446424055,-2.33759141173628E-5,
22.5540747194623));
#22644=CARTESIAN_POINT('Ctrl Pts',(-2.05801030910826,0.678835990556527,
22.5170984924742));
#22645=CARTESIAN_POINT('Ctrl Pts',(-1.31953539558407,2.03801862491187,22.4430778928222));
#22646=CARTESIAN_POINT('Ctrl Pts',(0.995655084428766,2.21510102422083,22.3320129205065));
#22647=CARTESIAN_POINT('Ctrl Pts',(2.40100336441846,0.364944432351608,22.2208798025149));
#22648=CARTESIAN_POINT('Ctrl Pts',(1.60885886272077,-1.81922366807872,22.1097466845233));
#22649=CARTESIAN_POINT('Ctrl Pts',(-0.655776594206566,-2.33836666353754,
21.9986135665318));
#22650=CARTESIAN_POINT('Ctrl Pts',(-1.93217795383359,-1.0952630718048,21.9133895781781));
#22651=CARTESIAN_POINT('Ctrl Pts',(-2.05508510116615,-0.207405785084765,
21.8652099624883));
#22652=CARTESIAN_POINT('Ctrl Pts',(-2.05341424816682,-0.0017536887259971,
21.8540747194623));
#22653=CARTESIAN_POINT('Origin',(0.,0.,30.5459252805377));
#22654=CARTESIAN_POINT('',(-2.05348239882457,0.00176844693486861,23.2540747194623));
#22655=CARTESIAN_POINT('',(-2.05448631486103,-0.00187785994470203,23.1959252805377));
#22656=CARTESIAN_POINT('',(-2.05475,1.58232769237955E-13,30.5459252805377));
#22657=CARTESIAN_POINT('Ctrl Pts',(-2.05448631486103,-0.00187785994470195,
23.1959252805377));
#22658=CARTESIAN_POINT('Ctrl Pts',(-2.04980780123993,0.513338964801136,
23.1679913295623));
#22659=CARTESIAN_POINT('Ctrl Pts',(-1.59250660598457,1.71920910668239,23.1030130059232));
#22660=CARTESIAN_POINT('Ctrl Pts',(0.43224489671947,2.38980469125578,23.0009903096202));
#22661=CARTESIAN_POINT('Ctrl Pts',(2.24219509588329,0.933039798232153,22.8898571916286));
#22662=CARTESIAN_POINT('Ctrl Pts',(2.00000009135574,-1.37767984222214,22.778724073637));
#22663=CARTESIAN_POINT('Ctrl Pts',(-0.072673716017103,-2.42749266612454,
22.6675909556455));
#22664=CARTESIAN_POINT('Ctrl Pts',(-1.77435552575201,-1.43343346508708,
22.573324691279));
#22665=CARTESIAN_POINT('Ctrl Pts',(-2.05068811746153,-0.373028609718886,
22.5161027995764));
#22666=CARTESIAN_POINT('Ctrl Pts',(-2.05149685129519,0.000497173714744739,
22.4959252805377));
#22667=CARTESIAN_POINT('Ctrl Pts',(-2.05348239882457,0.00176844693486848,
23.2540747194623));
#22668=CARTESIAN_POINT('Ctrl Pts',(-2.05515072772512,0.204886378054778,
23.2430757677879));
#22669=CARTESIAN_POINT('Ctrl Pts',(-1.93415066850296,1.09015999771089,23.1950324434495));
#22670=CARTESIAN_POINT('Ctrl Pts',(-0.664354069263913,2.33594419139362,
23.1099447464474));
#22671=CARTESIAN_POINT('Ctrl Pts',(1.60217141007485,1.82511598738049,22.9988116284558));
#22672=CARTESIAN_POINT('Ctrl Pts',(2.40232655406092,-0.356130204148507,
22.8876785104642));
#22673=CARTESIAN_POINT('Ctrl Pts',(1.00377788111867,-2.21143201569255,22.7765453924727));
#22674=CARTESIAN_POINT('Ctrl Pts',(-1.3134678169358,-2.04274420535881,22.6654122744811));
#22675=CARTESIAN_POINT('Ctrl Pts',(-2.0575570926931,-0.68263587599728,22.5912553834777));
#22676=CARTESIAN_POINT('Ctrl Pts',(-2.05812467462379,-0.00127448599310305,
22.5541428651381));
#22677=CARTESIAN_POINT('Ctrl Pts',(-2.05812446424055,-2.33759141173628E-5,
22.5540747194623));
#22678=CARTESIAN_POINT('Origin',(0.,0.,30.5459252805377));
#22679=CARTESIAN_POINT('',(-2.05188677382997,-0.0010204005874441,23.9540747194623));
#22680=CARTESIAN_POINT('',(-2.05787060010134,0.000654429798481389,23.8959252805377));
#22681=CARTESIAN_POINT('',(-2.05475,1.58232769237955E-13,30.5459252805377));
#22682=CARTESIAN_POINT('Ctrl Pts',(-2.05787060010134,0.000654429798481659,
23.8959252805377));
#22683=CARTESIAN_POINT('Ctrl Pts',(-2.05802039377806,0.0365895959979924,
23.893968604876));
#22684=CARTESIAN_POINT('Ctrl Pts',(-2.04088291558022,0.752714337046035,
23.8549675565504));
#22685=CARTESIAN_POINT('Ctrl Pts',(-1.20793243662604,2.10687003434831,23.7789221355611));
#22686=CARTESIAN_POINT('Ctrl Pts',(1.11489242455252,2.15754883948512,23.6677890175695));
#22687=CARTESIAN_POINT('Ctrl Pts',(2.4173238570424,0.233554026430338,23.556655899578));
#22688=CARTESIAN_POINT('Ctrl Pts',(1.50732535062721,-1.90419862421039,23.4455227815864));
#22689=CARTESIAN_POINT('Ctrl Pts',(-0.782236644429685,-2.29915374544626,
23.3343896635949));
#22690=CARTESIAN_POINT('Ctrl Pts',(-1.96032433113491,-1.01948053926428,
23.2511904965786));
#22691=CARTESIAN_POINT('Ctrl Pts',(-2.05601217248144,-0.169911466741311,
23.2050357022262));
#22692=CARTESIAN_POINT('Ctrl Pts',(-2.05448631486103,-0.00187785994470195,
23.1959252805377));
#22693=CARTESIAN_POINT('Ctrl Pts',(-2.05188677382997,-0.00102040058744382,
23.9540747194623));
#22694=CARTESIAN_POINT('Ctrl Pts',(-2.05005157165762,0.407271771044751,
23.9320086704376));
#22695=CARTESIAN_POINT('Ctrl Pts',(-1.73425658592992,1.50361854917053,23.8728982487491));
#22696=CARTESIAN_POINT('Ctrl Pts',(0.0508152693856986,2.42804847625626,
23.7767434543967));
#22697=CARTESIAN_POINT('Ctrl Pts',(2.06744504127525,1.27423412132916,23.6656103364052));
#22698=CARTESIAN_POINT('Ctrl Pts',(2.19186773754582,-1.04580945480468,23.5544772184136));
#22699=CARTESIAN_POINT('Ctrl Pts',(0.310206809340991,-2.40868705524225,
23.443344100422));
#22700=CARTESIAN_POINT('Ctrl Pts',(-1.64103861628355,-1.65033813069636,
23.343209934105));
#22701=CARTESIAN_POINT('Ctrl Pts',(-2.04953181063674,-0.479213030490258,
23.2801201404517));
#22702=CARTESIAN_POINT('Ctrl Pts',(-2.05348239882457,0.00176844693486848,
23.2540747194623));
#22703=CARTESIAN_POINT('Origin',(0.,0.,30.5459252805377));
#22704=CARTESIAN_POINT('',(-2.05720656193685,-0.00121771516567365,24.6540747194623));
#22705=CARTESIAN_POINT('',(-2.05255723160113,0.00146350343929692,24.5959252805377));
#22706=CARTESIAN_POINT('',(-2.05475,1.58232769237955E-13,30.5459252805377));
#22707=CARTESIAN_POINT('Ctrl Pts',(-2.05255723160113,0.00146350343929682,
24.5959252805377));
#22708=CARTESIAN_POINT('Ctrl Pts',(-2.05414229361448,0.242247432832211,
24.5829015075258));
#22709=CARTESIAN_POINT('Ctrl Pts',(-1.90365362879482,1.16599091497401,24.53283336185));
#22710=CARTESIAN_POINT('Ctrl Pts',(-0.536064276162042,2.36867836670812,
24.4457208435105));
#22711=CARTESIAN_POINT('Ctrl Pts',(1.69925433258817,1.73508986115085,24.3345877255189));
#22712=CARTESIAN_POINT('Ctrl Pts',(2.37934849415491,-0.486521177803125,
24.2234546075274));
#22713=CARTESIAN_POINT('Ctrl Pts',(0.881769263626921,-2.26284888554473,
24.1123214895357));
#22714=CARTESIAN_POINT('Ctrl Pts',(-1.38226358570042,-1.97331725525488,
24.0031450472059));
#22715=CARTESIAN_POINT('Ctrl Pts',(-2.05518445479657,-0.643745788400026,
23.9310129775398));
#22716=CARTESIAN_POINT('Ctrl Pts',(-2.05787060010134,0.000654429798481659,
23.8959252805377));
#22717=CARTESIAN_POINT('Ctrl Pts',(-2.05720656193685,-0.00121771516567365,
24.6540747194623));
#22718=CARTESIAN_POINT('Ctrl Pts',(-2.0529301797436,0.60780601961932,24.6209415730874));
#22719=CARTESIAN_POINT('Ctrl Pts',(-1.44395772496755,1.90517541785761,24.5507640540487));
#22720=CARTESIAN_POINT('Ctrl Pts',(0.761504884129454,2.30610318635139,24.4435421623461));
#22721=CARTESIAN_POINT('Ctrl Pts',(2.35045883035646,0.611019542610869,24.3324090443546));
#22722=CARTESIAN_POINT('Ctrl Pts',(1.7881803418832,-1.64329323602198,24.2212759263629));
#22723=CARTESIAN_POINT('Ctrl Pts',(-0.410711177573986,-2.39359936565602,
24.1101428083714));
#22724=CARTESIAN_POINT('Ctrl Pts',(-1.87173917948976,-1.23918996178022,
24.0210757394045));
#22725=CARTESIAN_POINT('Ctrl Pts',(-2.05313249987952,-0.278167083222276,
23.9690530431015));
#22726=CARTESIAN_POINT('Ctrl Pts',(-2.05188677382997,-0.00102040058744382,
23.9540747194623));
#22727=CARTESIAN_POINT('Origin',(0.,0.,30.5459252805377));
#22728=CARTESIAN_POINT('',(-2.05557731494487,0.00179379848086081,25.3540747194623));
#22729=CARTESIAN_POINT('',(-2.05258580046671,-0.00147696805610269,25.2959252805377));
#22730=CARTESIAN_POINT('',(-2.05475,1.58232769237955E-13,30.5459252805377));
#22731=CARTESIAN_POINT('Ctrl Pts',(-2.05258580046672,-0.00147696805610264,
25.2959252805377));
#22732=CARTESIAN_POINT('Ctrl Pts',(-2.04962418836947,0.443900223161274,
25.2718344101756));
#22733=CARTESIAN_POINT('Ctrl Pts',(-1.68833128126405,1.57850722809391,25.2106991671496));
#22734=CARTESIAN_POINT('Ctrl Pts',(0.183061725931824,2.4216710176215,25.1125195514598));
#22735=CARTESIAN_POINT('Ctrl Pts',(2.13381500276998,1.15967049071781,25.0013864334682));
#22736=CARTESIAN_POINT('Ctrl Pts',(2.13161680293297,-1.1637061134762,24.8902533154767));
#22737=CARTESIAN_POINT('Ctrl Pts',(0.178479005431905,-2.42201307959068,
24.7791201974851));
#22738=CARTESIAN_POINT('Ctrl Pts',(-1.68997690020491,-1.57591568347207,
24.6810108525055));
#22739=CARTESIAN_POINT('Ctrl Pts',(-2.04963379766141,-0.442630106399392,
24.6199458801896));
#22740=CARTESIAN_POINT('Ctrl Pts',(-2.05255723160113,0.00146350343929682,
24.5959252805377));
#22741=CARTESIAN_POINT('Ctrl Pts',(-2.05557731494487,0.00179379848086123,
25.3540747194623));
#22742=CARTESIAN_POINT('Ctrl Pts',(-2.05678373801941,0.13359791683739,25.3469188484011));
#22743=CARTESIAN_POINT('Ctrl Pts',(-1.98518594980207,0.946417566930667,
25.3027186046759));
#22744=CARTESIAN_POINT('Ctrl Pts',(-0.902106643086596,2.25481821865058,
25.221473988287));
#22745=CARTESIAN_POINT('Ctrl Pts',(1.40506247979517,1.98085865788643,25.1103408702954));
#22746=CARTESIAN_POINT('Ctrl Pts',(2.42626311844678,-0.106060712410309,
24.9992077523039));
#22747=CARTESIAN_POINT('Ctrl Pts',(1.22685225431082,-2.09590914420127,24.8880746343123));
#22748=CARTESIAN_POINT('Ctrl Pts',(-1.09542208140494,-2.16749903303861,
24.7769415163207));
#22749=CARTESIAN_POINT('Ctrl Pts',(-2.0216683440278,-0.825407580955758,
24.6989415447041));
#22750=CARTESIAN_POINT('Ctrl Pts',(-2.0577113705737,-0.0731103635467968,
24.6579859457513));
#22751=CARTESIAN_POINT('Ctrl Pts',(-2.05720656193685,-0.00121771516567365,
24.6540747194623));
#22752=CARTESIAN_POINT('Origin',(0.,0.,30.5459252805377));
#22753=CARTESIAN_POINT('',(-2.05138931231396,9.0883460209662E-5,26.0540747194623));
#22754=CARTESIAN_POINT('',(-2.05788771163865,-0.000632027364112667,25.9959252805377));
#22755=CARTESIAN_POINT('',(-2.05475,1.58232769237955E-13,30.5459252805377));
#22756=CARTESIAN_POINT('Ctrl Pts',(-2.05788771163865,-0.000632027364112779,
25.9959252805377));
#22757=CARTESIAN_POINT('Ctrl Pts',(-2.05527788428679,0.645044426388679,
25.9607673128253));
#22758=CARTESIAN_POINT('Ctrl Pts',(-1.37998469315385,1.97574570518029,25.8885649724492));
#22759=CARTESIAN_POINT('Ctrl Pts',(0.886049547518136,2.26117631167387,25.7793182594091));
#22760=CARTESIAN_POINT('Ctrl Pts',(2.38026485126002,0.482017998562706,25.6681851414176));
#22761=CARTESIAN_POINT('Ctrl Pts',(1.69596807681793,-1.73830215885906,25.557052023426));
#22762=CARTESIAN_POINT('Ctrl Pts',(-0.540545434181373,-2.36765976159588,
25.4459189054345));
#22763=CARTESIAN_POINT('Ctrl Pts',(-1.9047552100369,-1.16335890299012,25.358876657805));
#22764=CARTESIAN_POINT('Ctrl Pts',(-2.0541782397826,-0.240953349974224,
25.3088787828394));
#22765=CARTESIAN_POINT('Ctrl Pts',(-2.05258580046672,-0.00147696805610264,
25.2959252805377));
#22766=CARTESIAN_POINT('Ctrl Pts',(-2.05138931231396,9.08834602098355E-5,
26.0540747194623));
#22767=CARTESIAN_POINT('Ctrl Pts',(-2.05152243725439,0.337478144257027,
26.0358517510509));
#22768=CARTESIAN_POINT('Ctrl Pts',(-1.81315796563237,1.3605424797094,25.9805844099755));
#22769=CARTESIAN_POINT('Ctrl Pts',(-0.200277927177756,2.42030790331167,
25.8882726962363));
#22770=CARTESIAN_POINT('Ctrl Pts',(1.92475392154391,1.48098748682692,25.7771395782448));
#22771=CARTESIAN_POINT('Ctrl Pts',(2.28817522362595,-0.813790968595164,
25.6660064602532));
#22772=CARTESIAN_POINT('Ctrl Pts',(0.557368499380946,-2.36375589911376,
25.5548733422617));
#22773=CARTESIAN_POINT('Ctrl Pts',(-1.53926998825786,-1.78981768810613,
25.4508960953314));
#22774=CARTESIAN_POINT('Ctrl Pts',(-2.05053835075894,-0.548723052508241,
25.3839632210649));
#22775=CARTESIAN_POINT('Ctrl Pts',(-2.05557731494487,0.00179379848086123,
25.3540747194623));
#22776=CARTESIAN_POINT('Origin',(0.,0.,30.5459252805377));
#22777=CARTESIAN_POINT('',(-2.05524375550136,-0.00184130802409817,26.7540747194623));
#22778=CARTESIAN_POINT('',(-2.05444749037063,0.00187707957529171,26.6959252805377));
#22779=CARTESIAN_POINT('',(-2.05475,1.58232769237955E-13,30.5459252805377));
#22780=CARTESIAN_POINT('Ctrl Pts',(-2.05444749037063,0.00187707957529195,
26.6959252805377));
#22781=CARTESIAN_POINT('Ctrl Pts',(-2.05598194935013,0.171214930317575,
26.686744588139));
#22782=CARTESIAN_POINT('Ctrl Pts',(-1.95938878154241,1.02210918950486,26.6405195230765));
#22783=CARTESIAN_POINT('Ctrl Pts',(-0.777884683860044,2.30062981105139,
26.5572500853501));
#22784=CARTESIAN_POINT('Ctrl Pts',(1.51092586075795,1.90134298806969,26.4461169673585));
#22785=CARTESIAN_POINT('Ctrl Pts',(2.4168775880718,-0.238127775426892,26.3349838493669));
#22786=CARTESIAN_POINT('Ctrl Pts',(1.11080781944703,-2.15965462534927,26.2238507313753));
#22787=CARTESIAN_POINT('Ctrl Pts',(-1.21191698652597,-2.10458055943487,
26.1127176133838));
#22788=CARTESIAN_POINT('Ctrl Pts',(-2.04153625209659,-0.750103919255093,
26.0367424631046));
#22789=CARTESIAN_POINT('Ctrl Pts',(-2.05802774223653,-0.0352758745116443,
25.9978116854892));
#22790=CARTESIAN_POINT('Ctrl Pts',(-2.05788771163865,-0.000632027364112779,
25.9959252805377));
#22791=CARTESIAN_POINT('Ctrl Pts',(-2.05524375550136,-0.00184130802409798,
26.7540747194623));
#22792=CARTESIAN_POINT('Ctrl Pts',(-2.05026254246359,0.537878244060909,
26.7247846537006));
#22793=CARTESIAN_POINT('Ctrl Pts',(-1.55589885109608,1.76827887673406,26.6584502152751));
#22794=CARTESIAN_POINT('Ctrl Pts',(0.51920669687721,2.37243040203942,26.5550714041857));
#22795=CARTESIAN_POINT('Ctrl Pts',(2.27476474931693,0.850556836234861,26.4439382861941));
#22796=CARTESIAN_POINT('Ctrl Pts',(1.9483685659561,-1.44977981832677,26.3328051682026));
#22797=CARTESIAN_POINT('Ctrl Pts',(-0.161251214260656,-2.42322092316419,
26.221672050211));
#22798=CARTESIAN_POINT('Ctrl Pts',(-1.8015641250331,-1.38288211781774,26.1287619006309));
#22799=CARTESIAN_POINT('Ctrl Pts',(-2.05125181559754,-0.348376055716531,
26.0728961237147));
#22800=CARTESIAN_POINT('Ctrl Pts',(-2.05138931231396,9.08834602098355E-5,
26.0540747194623));
#22801=CARTESIAN_POINT('Origin',(0.,0.,30.5459252805377));
#22802=CARTESIAN_POINT('',(-2.05744477280677,0.00105931724472513,27.4540747194623));
#22803=CARTESIAN_POINT('',(-2.05150643897842,-0.000517795507161443,27.3959252805377));
#22804=CARTESIAN_POINT('',(-2.05475,1.58232769237955E-13,30.5459252805377));
#22805=CARTESIAN_POINT('Ctrl Pts',(-2.05150643897842,-0.000517795507161516,
27.3959252805377));
#22806=CARTESIAN_POINT('Ctrl Pts',(-2.05066106742218,0.374304485575549,
27.3756774907888));
#22807=CARTESIAN_POINT('Ctrl Pts',(-1.77290985721247,1.4360498631238,27.318385328376));
#22808=CARTESIAN_POINT('Ctrl Pts',(-0.0680801792595378,2.42762578972398,
27.2240487932994));
#22809=CARTESIAN_POINT('Ctrl Pts',(2.00260341844735,1.37389291172196,27.1129156753079));
#22810=CARTESIAN_POINT('Ctrl Pts',(2.24042554204435,-0.937280921003925,
27.0017825573163));
#22811=CARTESIAN_POINT('Ctrl Pts',(0.427722029271838,-2.39061831907088,
26.8906494393248));
#22812=CARTESIAN_POINT('Ctrl Pts',(-1.59436319612448,-1.716657147866,26.7886970137318));
#22813=CARTESIAN_POINT('Ctrl Pts',(-2.04979036076342,-0.512068440541057,
26.7237889608028));
#22814=CARTESIAN_POINT('Ctrl Pts',(-2.05444749037063,0.00187707957529195,
26.6959252805377));
#22815=CARTESIAN_POINT('Ctrl Pts',(-2.05744477280677,0.00105931724472533,
27.4540747194623));
#22816=CARTESIAN_POINT('Ctrl Pts',(-2.05782716792171,0.061933506835561,
27.4507619290143));
#22817=CARTESIAN_POINT('Ctrl Pts',(-2.02776705731346,0.803133697963998,
27.4104047659024));
#22818=CARTESIAN_POINT('Ctrl Pts',(-1.13020663702663,2.14956575456656,27.3330032301266));
#22819=CARTESIAN_POINT('Ctrl Pts',(1.19291950474651,2.1154065927935,27.2218701121351));
#22820=CARTESIAN_POINT('Ctrl Pts',(2.42423908872827,0.145143535993706,27.1107369941435));
#22821=CARTESIAN_POINT('Ctrl Pts',(1.43679947210715,-1.95796032739892,26.999603876152));
#22822=CARTESIAN_POINT('Ctrl Pts',(-0.865655485103571,-2.26906197521519,
26.8884707581604));
#22823=CARTESIAN_POINT('Ctrl Pts',(-1.97780974213485,-0.968776180348794,
26.8066277059305));
#22824=CARTESIAN_POINT('Ctrl Pts',(-2.05656249117625,-0.144727673729697,
26.7618290263645));
#22825=CARTESIAN_POINT('Ctrl Pts',(-2.05524375550136,-0.00184130802409798,
26.7540747194623));
#22826=CARTESIAN_POINT('Origin',(0.,0.,30.5459252805377));
#22827=CARTESIAN_POINT('',(-2.05206134370476,0.00116288414692314,28.1540747194623));
#22828=CARTESIAN_POINT('',(-2.05634566411282,-0.00160712594267666,28.0959252805377));
#22829=CARTESIAN_POINT('',(-2.05475,1.58232769237955E-13,30.5459252805377));
#22830=CARTESIAN_POINT('Ctrl Pts',(-2.05634566411282,-0.00160712594267667,
28.0959252805377));
#22831=CARTESIAN_POINT('Ctrl Pts',(-2.05139599927139,0.574624822876943,
28.0646103934386));
#22832=CARTESIAN_POINT('Ctrl Pts',(-1.49844858220422,1.84084696248835,27.9962511336756));
#22833=CARTESIAN_POINT('Ctrl Pts',(0.647725970766636,2.34060717669366,27.8908475012488));
#22834=CARTESIAN_POINT('Ctrl Pts',(2.31773743276476,0.725325684108574,27.7797143832572));
#22835=CARTESIAN_POINT('Ctrl Pts',(1.86646417683138,-1.55380676849557,27.6685812652656));
#22836=CARTESIAN_POINT('Ctrl Pts',(-0.293070456042677,-2.41083184926652,
27.5574481472741));
#22837=CARTESIAN_POINT('Ctrl Pts',(-1.83979104753125,-1.30723380638585,
27.4665628190314));
#22838=CARTESIAN_POINT('Ctrl Pts',(-2.05220771816071,-0.311452154301391,
27.4127218634526));
#22839=CARTESIAN_POINT('Ctrl Pts',(-2.05150643897842,-0.000517795507161516,
27.3959252805377));
#22840=CARTESIAN_POINT('Ctrl Pts',(-2.05206134370476,0.00116288414692349,
28.1540747194623));
#22841=CARTESIAN_POINT('Ctrl Pts',(-2.05344175345948,0.26718383829129,28.1396948316641));
#22842=CARTESIAN_POINT('Ctrl Pts',(-1.8817859926555,1.21680050673287,28.0882705712019));
#22843=CARTESIAN_POINT('Ctrl Pts',(-0.449219217968869,2.38665611117453,
27.999801938076));
#22844=CARTESIAN_POINT('Ctrl Pts',(1.76146356868064,1.6719019509933,27.8886688200844));
#22845=CARTESIAN_POINT('Ctrl Pts',(2.36000201199169,-0.573068912759941,
27.7775357020928));
#22846=CARTESIAN_POINT('Ctrl Pts',(0.798565170672349,-2.29353090612058,
27.6664025841013));
#22847=CARTESIAN_POINT('Ctrl Pts',(-1.42541352622956,-1.92615781520145,
27.5585822565578));
#22848=CARTESIAN_POINT('Ctrl Pts',(-2.05355113918859,-0.618775460476319,
27.4878063016781));
#22849=CARTESIAN_POINT('Ctrl Pts',(-2.05744477280677,0.00105931724472533,
27.4540747194623));
#22850=CARTESIAN_POINT('Origin',(0.,0.,30.5459252805377));
#22851=CARTESIAN_POINT('',(-2.05269153525815,-0.00250469671298922,28.8540747194623));
#22852=CARTESIAN_POINT('',(-2.05654741388298,0.00148211099959903,28.7959252805377));
#22853=CARTESIAN_POINT('',(-2.05475,1.58232769237955E-13,30.5459252805377));
#22854=CARTESIAN_POINT('',(-0.530170217188662,-1.98517432567171,29.));
#22855=CARTESIAN_POINT('Ctrl Pts',(-0.530170217188634,-1.98517432567172,
29.));
#22856=CARTESIAN_POINT('Ctrl Pts',(-1.19025956241812,-1.80888768575368,
28.9629556273361));
#22857=CARTESIAN_POINT('Ctrl Pts',(-1.92498012557237,-1.11310439800918,
28.9143138671569));
#22858=CARTESIAN_POINT('Ctrl Pts',(-2.05431617558531,-0.216806977145675,
28.8656721069777));
#22859=CARTESIAN_POINT('Ctrl Pts',(-2.05269153525815,-0.00250469671298928,
28.8540747194623));
#22860=CARTESIAN_POINT('',(0.531258132123393,-1.9887550962016,29.));
#22861=CARTESIAN_POINT('Origin',(0.,0.,29.));
#22862=CARTESIAN_POINT('Ctrl Pts',(0.53125844574167,-1.98875612844696,29.));
#22863=CARTESIAN_POINT('Ctrl Pts',(-0.113293144729996,-2.16008022379809,
28.9636818543909));
#22864=CARTESIAN_POINT('Ctrl Pts',(-1.49287139477788,-1.84060537719605,
28.8956569479035));
#22865=CARTESIAN_POINT('Ctrl Pts',(-2.05167852337285,-0.581660892242976,
28.8276320414161));
#22866=CARTESIAN_POINT('Ctrl Pts',(-2.05654741388298,0.00148211099959938,
28.7959252805377));
#22867=CARTESIAN_POINT('Origin',(-4.61329551933804E-17,0.,18.));
#22868=CARTESIAN_POINT('Ctrl Pts',(-0.76990204067047,-1.47743251885541,
18.));
#22869=CARTESIAN_POINT('Ctrl Pts',(-0.718150631325321,-1.51251203856552,
18.));
#22870=CARTESIAN_POINT('Ctrl Pts',(-0.664423318055599,-1.5443372549372,
18.));
#22871=CARTESIAN_POINT('Ctrl Pts',(-0.609051292693035,-1.57297177961208,
18.));
#22872=CARTESIAN_POINT('Ctrl Pts',(-0.5739254652649,-1.59113639189834,18.));
#22873=CARTESIAN_POINT('Ctrl Pts',(-0.538136890245182,-1.60801638025237,
18.));
#22874=CARTESIAN_POINT('Ctrl Pts',(-0.501762501547232,-1.62362076387509,
18.));
#22875=CARTESIAN_POINT('Ctrl Pts',(-0.476746252182073,-1.63435257727097,
18.));
#22876=CARTESIAN_POINT('Ctrl Pts',(-0.45145279912961,-1.64448092345754,
18.));
#22877=CARTESIAN_POINT('Ctrl Pts',(-0.425905888015268,-1.65400710125167,
18.));
#22878=CARTESIAN_POINT('Ctrl Pts',(-0.41253154468577,-1.65899425495751,
18.));
#22879=CARTESIAN_POINT('Ctrl Pts',(-0.399088138260695,-1.66381606897088,
18.));
#22880=CARTESIAN_POINT('Ctrl Pts',(-0.385592178738817,-1.66846843086131,
18.));
#22881=CARTESIAN_POINT('Ctrl Pts',(-0.323215765718591,-1.68997098844724,
18.));
#22882=CARTESIAN_POINT('Ctrl Pts',(-0.259649271127304,-1.70788387774854,
18.));
#22883=CARTESIAN_POINT('Ctrl Pts',(-0.195242368079891,-1.72225306016113,
18.));
#22884=CARTESIAN_POINT('Ctrl Pts',(-0.148812097770522,-1.73261165515598,
18.));
#22885=CARTESIAN_POINT('Ctrl Pts',(-0.101944183746803,-1.74112782318747,
18.));
#22886=CARTESIAN_POINT('Ctrl Pts',(-0.0547605417505049,-1.7478047767719,
18.));
#22887=CARTESIAN_POINT('Ctrl Pts',(-0.0416678989315785,-1.7496575156598,
18.));
#22888=CARTESIAN_POINT('Ctrl Pts',(-0.0285509121040071,-1.75136856900838,
18.));
#22889=CARTESIAN_POINT('Ctrl Pts',(-0.0154121163252258,-1.75293783687761,
18.));
#22890=CARTESIAN_POINT('Ctrl Pts',(-0.00237504775858612,-1.75449495468012,
18.));
#22891=CARTESIAN_POINT('Ctrl Pts',(0.0106749433642533,-1.75591142474928,
18.));
#22892=CARTESIAN_POINT('Ctrl Pts',(0.0237314174192055,-1.75718732825168,
18.));
#22893=CARTESIAN_POINT('Ctrl Pts',(0.091264839179258,-1.76378682280057,
18.));
#22894=CARTESIAN_POINT('Ctrl Pts',(0.159001654673738,-1.76663304455511,
18.));
#22895=CARTESIAN_POINT('Ctrl Pts',(0.226587398060141,-1.76577341924289,
18.));
#22896=CARTESIAN_POINT('Ctrl Pts',(0.295141384080251,-1.7649014788205,18.));
#22897=CARTESIAN_POINT('Ctrl Pts',(0.363540948302614,-1.76021708355991,
18.));
#22898=CARTESIAN_POINT('Ctrl Pts',(0.431437640562689,-1.75172144275485,
18.));
#22899=CARTESIAN_POINT('Ctrl Pts',(0.473486932876576,-1.74645998344492,
18.));
#22900=CARTESIAN_POINT('Ctrl Pts',(0.51534371614305,-1.73973575700245,18.));
#22901=CARTESIAN_POINT('Ctrl Pts',(0.556926593833155,-1.73153911679675,
18.));
#22902=CARTESIAN_POINT('Ctrl Pts',(0.591007346597968,-1.72482126358721,
18.));
#22903=CARTESIAN_POINT('Ctrl Pts',(0.624904151165585,-1.71711422326624,
18.));
#22904=CARTESIAN_POINT('Ctrl Pts',(0.658571851627645,-1.70840869390865,
18.));
#22905=CARTESIAN_POINT('Ctrl Pts',(0.672311891199144,-1.70485590247287,
18.));
#22906=CARTESIAN_POINT('Ctrl Pts',(0.686016147209164,-1.70113595255256,
18.));
#22907=CARTESIAN_POINT('Ctrl Pts',(0.699658483569614,-1.69725500100484,
18.));
#22908=CARTESIAN_POINT('Ctrl Pts',(0.767448475183213,-1.67797020506366,
18.));
#22909=CARTESIAN_POINT('Ctrl Pts',(0.833829915647279,-1.65468448734625,
18.));
#22910=CARTESIAN_POINT('Ctrl Pts',(0.898440425741411,-1.62741601672657,
18.));
#22911=CARTESIAN_POINT('Ctrl Pts',(0.905588436264334,-1.62439924260346,
18.));
#22912=CARTESIAN_POINT('Ctrl Pts',(0.912714779380887,-1.62133366961292,
18.));
#22913=CARTESIAN_POINT('Ctrl Pts',(0.919818968510682,-1.61821928330016,
18.));
#22914=CARTESIAN_POINT('Ctrl Pts',(0.981562897597664,-1.5911515287498,18.));
#22915=CARTESIAN_POINT('Ctrl Pts',(1.04163420093584,-1.56040088867233,18.));
#22916=CARTESIAN_POINT('Ctrl Pts',(1.09989073176884,-1.52627787643936,18.));
#22917=CARTESIAN_POINT('Ctrl Pts',(1.16256978924498,-1.48956442621451,18.));
#22918=CARTESIAN_POINT('Ctrl Pts',(1.22314908610384,-1.44894713491801,18.));
#22919=CARTESIAN_POINT('Ctrl Pts',(1.28143172127969,-1.40475162384861,18.));
#22920=CARTESIAN_POINT('Ctrl Pts',(1.29192404292766,-1.3967953343614,18.));
#22921=CARTESIAN_POINT('Ctrl Pts',(1.30234185924819,-1.38872293100869,18.));
#22922=CARTESIAN_POINT('Ctrl Pts',(1.31268391753456,-1.38053612650623,18.));
#22923=CARTESIAN_POINT('Ctrl Pts',(1.32189334531869,-1.37324591572222,18.));
#22924=CARTESIAN_POINT('Ctrl Pts',(1.33103577871284,-1.36587044480612,18.));
#22925=CARTESIAN_POINT('Ctrl Pts',(1.34010835513525,-1.35841319152643,18.));
#22926=CARTESIAN_POINT('Ctrl Pts',(1.39501139656529,-1.31328533955731,18.));
#22927=CARTESIAN_POINT('Ctrl Pts',(1.44738363710458,-1.26514600652793,18.));
#22928=CARTESIAN_POINT('Ctrl Pts',(1.49707481635619,-1.21434556759909,18.));
#22929=CARTESIAN_POINT('Ctrl Pts',(1.54781663370407,-1.16247103710612,18.));
#22930=CARTESIAN_POINT('Ctrl Pts',(1.59576358322206,-1.10782114035041,18.));
#22931=CARTESIAN_POINT('Ctrl Pts',(1.64073548547958,-1.0507176415564,18.));
#22932=CARTESIAN_POINT('Ctrl Pts',(1.68598205390614,-0.993265382793032,
18.));
#22933=CARTESIAN_POINT('Ctrl Pts',(1.72821791230343,-0.933328730063129,
18.));
#22934=CARTESIAN_POINT('Ctrl Pts',(1.76722761838473,-0.871193823462839,
18.));
#22935=CARTESIAN_POINT('Ctrl Pts',(1.7768492490117,-0.85586842933904,18.));
#22936=CARTESIAN_POINT('Ctrl Pts',(1.78627443371382,-0.840409138082932,
18.));
#22937=CARTESIAN_POINT('Ctrl Pts',(1.79549955621922,-0.824819938514783,
18.));
#22938=CARTESIAN_POINT('Ctrl Pts',(1.80276226427272,-0.812546951875862,
18.));
#22939=CARTESIAN_POINT('Ctrl Pts',(1.80990173580295,-0.800191855082187,
18.));
#22940=CARTESIAN_POINT('Ctrl Pts',(1.81690568883513,-0.787775762904653,
18.));
#22941=CARTESIAN_POINT('Ctrl Pts',(1.85392851007218,-0.722144431706478,
18.));
#22942=CARTESIAN_POINT('Ctrl Pts',(1.8872372067062,-0.654696535289144,18.));
#22943=CARTESIAN_POINT('Ctrl Pts',(1.91665075707102,-0.585778873556434,
18.));
#22944=CARTESIAN_POINT('Ctrl Pts',(1.94609703420479,-0.516784531097881,
18.));
#22945=CARTESIAN_POINT('Ctrl Pts',(1.97164025822083,-0.446316320651974,
18.));
#22946=CARTESIAN_POINT('Ctrl Pts',(1.99306307145695,-0.374684480774626,
18.));
#22947=CARTESIAN_POINT('Ctrl Pts',(2.01399797892016,-0.304684060067817,
18.));
#22948=CARTESIAN_POINT('Ctrl Pts',(2.03099858110164,-0.233571531454558,
18.));
#22949=CARTESIAN_POINT('Ctrl Pts',(2.04381843104347,-0.161613213448295,
18.));
#22950=CARTESIAN_POINT('Ctrl Pts',(2.0465707882259,-0.146164125175105,18.));
#22951=CARTESIAN_POINT('Ctrl Pts',(2.04913025745793,-0.130675991664333,
18.));
#22952=CARTESIAN_POINT('Ctrl Pts',(2.05149409115388,-0.115151364067968,
18.));
#22953=CARTESIAN_POINT('Ctrl Pts',(2.05350777753846,-0.101926351128162,
18.));
#22954=CARTESIAN_POINT('Ctrl Pts',(2.05537949127336,-0.0886748543274951,
18.));
#22955=CARTESIAN_POINT('Ctrl Pts',(2.0571100610898,-0.075398570255039,18.));
#22956=CARTESIAN_POINT('Ctrl Pts',(1.81742788875943,0.958620587959298,18.));
#22957=CARTESIAN_POINT('Ctrl Pts',(1.77657712986193,1.02110689942424,18.));
#22958=CARTESIAN_POINT('Ctrl Pts',(1.7321315874396,1.08104302965111,18.));
#22959=CARTESIAN_POINT('Ctrl Pts',(1.68441962095058,1.13827891073254,18.));
#22960=CARTESIAN_POINT('Ctrl Pts',(1.63796461382492,1.19400692739462,18.));
#22961=CARTESIAN_POINT('Ctrl Pts',(1.58841202635459,1.24717530230443,18.));
#22962=CARTESIAN_POINT('Ctrl Pts',(1.5360388941578,1.29760785240109,18.));
#22963=CARTESIAN_POINT('Ctrl Pts',(1.52434810361592,1.3088654639844,18.));
#22964=CARTESIAN_POINT('Ctrl Pts',(1.51251510017348,1.3199880593865,18.));
#22965=CARTESIAN_POINT('Ctrl Pts',(1.50054796988442,1.33096871964239,18.));
#22966=CARTESIAN_POINT('Ctrl Pts',(1.44563515565536,1.38135498119215,18.));
#22967=CARTESIAN_POINT('Ctrl Pts',(1.38801000276354,1.42865729042352,18.));
#22968=CARTESIAN_POINT('Ctrl Pts',(1.32798805944486,1.47270290942279,18.));
#22969=CARTESIAN_POINT('Ctrl Pts',(1.28585164904722,1.5036236723264,18.));
#22970=CARTESIAN_POINT('Ctrl Pts',(1.24253335224023,1.53293855420436,18.));
#22971=CARTESIAN_POINT('Ctrl Pts',(1.19813701502426,1.56057339033618,18.));
#22972=CARTESIAN_POINT('Ctrl Pts',(1.18125759993015,1.57108011002022,18.));
#22973=CARTESIAN_POINT('Ctrl Pts',(1.16422232469794,1.58134384847995,18.));
#22974=CARTESIAN_POINT('Ctrl Pts',(1.14703682092037,1.59136004184456,18.));
#22975=CARTESIAN_POINT('Ctrl Pts',(1.13066871649995,1.60089983194957,18.));
#22976=CARTESIAN_POINT('Ctrl Pts',(1.11415903455404,1.61021779338036,18.));
#22977=CARTESIAN_POINT('Ctrl Pts',(1.09754217891543,1.61929409944754,18.));
#22978=CARTESIAN_POINT('Ctrl Pts',(1.03383800288656,1.65409000861173,18.));
#22979=CARTESIAN_POINT('Ctrl Pts',(0.96849489309373,1.68537885814686,18.));
#22980=CARTESIAN_POINT('Ctrl Pts',(0.901803973692338,1.71299878952967,18.));
#22981=CARTESIAN_POINT('Ctrl Pts',(0.836547032382178,1.74002484131329,18.));
#22982=CARTESIAN_POINT('Ctrl Pts',(0.769998695925455,1.76353820983274,18.));
#22983=CARTESIAN_POINT('Ctrl Pts',(0.702423095374045,1.78333899888662,18.));
#22984=CARTESIAN_POINT('Ctrl Pts',(0.63632849633975,1.8027058295533,18.));
#22985=CARTESIAN_POINT('Ctrl Pts',(0.569250406487646,1.81852114051121,18.));
#22986=CARTESIAN_POINT('Ctrl Pts',(0.501439873296343,1.83054930271628,18.));
#22987=CARTESIAN_POINT('Ctrl Pts',(0.479368946632993,1.83446422084816,18.));
#22988=CARTESIAN_POINT('Ctrl Pts',(0.457220505887409,1.83797754309986,18.));
#22989=CARTESIAN_POINT('Ctrl Pts',(0.435003501016378,1.8410799689604,18.));
#22990=CARTESIAN_POINT('Ctrl Pts',(0.422525526393832,1.84282241765593,18.));
#22991=CARTESIAN_POINT('Ctrl Pts',(0.410024644591693,1.8444352959301,18.));
#22992=CARTESIAN_POINT('Ctrl Pts',(0.397520124711553,1.84591507854722,18.));
#22993=CARTESIAN_POINT('Ctrl Pts',(0.329697086251002,1.85394124463088,18.));
#22994=CARTESIAN_POINT('Ctrl Pts',(0.261648673649785,1.85807376866092,18.));
#22995=CARTESIAN_POINT('Ctrl Pts',(0.193620068644232,1.85813442656068,18.));
#22996=CARTESIAN_POINT('Ctrl Pts',(0.183819205913209,1.8581431655279,18.));
#22997=CARTESIAN_POINT('Ctrl Pts',(0.174018760470502,1.85806730026065,18.));
#22998=CARTESIAN_POINT('Ctrl Pts',(0.164219474866952,1.85790620769987,18.));
#22999=CARTESIAN_POINT('Ctrl Pts',(0.0948546883628424,1.85676590507598,
18.));
#23000=CARTESIAN_POINT('Ctrl Pts',(0.0255465610762253,1.85135924381112,
18.));
#23001=CARTESIAN_POINT('Ctrl Pts',(-0.0433793899519713,1.84185967358528,
18.));
#23002=CARTESIAN_POINT('Ctrl Pts',(-0.107679490493548,1.83299765120457,
18.));
#23003=CARTESIAN_POINT('Ctrl Pts',(-0.171647506113411,1.82057273856315,
18.));
#23004=CARTESIAN_POINT('Ctrl Pts',(-0.234998654721344,1.80469130867306,
18.));
#23005=CARTESIAN_POINT('Ctrl Pts',(-0.248859420949268,1.80121656840538,
18.));
#23006=CARTESIAN_POINT('Ctrl Pts',(-0.262690559254527,1.79757625312175,
18.));
#23007=CARTESIAN_POINT('Ctrl Pts',(-0.276488909329196,1.79377129906237,
18.));
#23008=CARTESIAN_POINT('Ctrl Pts',(-0.287551928784525,1.79072062412242,
18.));
#23009=CARTESIAN_POINT('Ctrl Pts',(-0.298593335771869,1.7875641728674,18.));
#23010=CARTESIAN_POINT('Ctrl Pts',(-0.309598430415198,1.78430655809845,
18.));
#23011=CARTESIAN_POINT('Ctrl Pts',(-0.375170595375803,1.7648965611897,18.));
#23012=CARTESIAN_POINT('Ctrl Pts',(-0.439577642441152,1.74186598076745,
18.));
#23013=CARTESIAN_POINT('Ctrl Pts',(-0.502516607245069,1.7153970604683,18.));
#23014=CARTESIAN_POINT('Ctrl Pts',(-0.565162708177599,1.68905130378479,
18.));
#23015=CARTESIAN_POINT('Ctrl Pts',(-0.626355250869692,1.65929842798695,
18.));
#23016=CARTESIAN_POINT('Ctrl Pts',(-0.685765693704282,1.62627659429092,
18.));
#23017=CARTESIAN_POINT('Ctrl Pts',(-0.743900118729632,1.59396400371579,
18.));
#23018=CARTESIAN_POINT('Ctrl Pts',(-0.800328846584056,1.55852066563614,
18.));
#23019=CARTESIAN_POINT('Ctrl Pts',(-0.854704114065593,1.52004664194688,
18.));
#23020=CARTESIAN_POINT('Ctrl Pts',(-0.866188890450393,1.511920418773,18.));
#23021=CARTESIAN_POINT('Ctrl Pts',(-0.877581894981679,1.50365890819555,
18.));
#23022=CARTESIAN_POINT('Ctrl Pts',(-0.888879573567156,1.49526292491495,
18.));
#23023=CARTESIAN_POINT('Ctrl Pts',(-0.899528318420504,1.48734920325332,
18.));
#23024=CARTESIAN_POINT('Ctrl Pts',(-0.910093638757256,1.47931487609194,
18.));
#23025=CARTESIAN_POINT('Ctrl Pts',(-0.92055590532325,1.47117394178587,18.));
#23026=CARTESIAN_POINT('Ctrl Pts',(-0.972133500375775,1.43104020878076,
18.));
#23027=CARTESIAN_POINT('Ctrl Pts',(-1.02130427170992,1.38824940731442,18.));
#23028=CARTESIAN_POINT('Ctrl Pts',(-1.06777672763296,1.34293373535765,18.));
#23029=CARTESIAN_POINT('Ctrl Pts',(-1.11336328516427,1.29848191017009,18.));
#23030=CARTESIAN_POINT('Ctrl Pts',(-1.15635400485184,1.25159989688763,18.));
#23031=CARTESIAN_POINT('Ctrl Pts',(-1.19643122999363,1.20238672968345,18.));
#23032=CARTESIAN_POINT('Ctrl Pts',(-1.23520491944242,1.15477425014636,18.));
#23033=CARTESIAN_POINT('Ctrl Pts',(-1.27125189947612,1.10497922195428,18.));
#23034=CARTESIAN_POINT('Ctrl Pts',(-1.30423784606576,1.05307598279351,18.));
#23035=CARTESIAN_POINT('Ctrl Pts',(-1.30970514760245,1.0444732083225,18.));
#23036=CARTESIAN_POINT('Ctrl Pts',(-1.31508824330323,1.03581249296888,18.));
#23037=CARTESIAN_POINT('Ctrl Pts',(-1.32038547188529,1.02709414911752,18.));
#23038=CARTESIAN_POINT('Ctrl Pts',(-1.32604175486339,1.01778486235373,18.));
#23039=CARTESIAN_POINT('Ctrl Pts',(-1.33160013514927,1.00840986902262,18.));
#23040=CARTESIAN_POINT('Ctrl Pts',(-1.33706021092902,0.998970828965279,
18.));
#23041=CARTESIAN_POINT('Origin',(0.,0.,30.5459252805377));
#23042=CARTESIAN_POINT('Ctrl Pts',(-2.05654741388298,0.0014821109995993,
28.7959252805377));
#23043=CARTESIAN_POINT('Ctrl Pts',(-2.05736705760088,0.0996501635064194,
28.7905876687522));
#23044=CARTESIAN_POINT('Ctrl Pts',(-2.00636102311651,0.87830624679129,28.7482056843029));
#23045=CARTESIAN_POINT('Ctrl Pts',(-1.01137155273683,2.20819495159188,28.6687793271897));
#23046=CARTESIAN_POINT('Ctrl Pts',(1.30642536602,2.04713238573498,28.5576462091981));
#23047=CARTESIAN_POINT('Ctrl Pts',(2.428549244938,0.0128757876891458,28.4465130912066));
#23048=CARTESIAN_POINT('Ctrl Pts',(1.32795945590719,-2.03338475909482,28.335379973215));
#23049=CARTESIAN_POINT('Ctrl Pts',(-0.988025992283097,-2.21849736833443,
28.2242468552234));
#23050=CARTESIAN_POINT('Ctrl Pts',(-2.00194536412696,-0.89317403920961,
28.144428624331));
#23051=CARTESIAN_POINT('Ctrl Pts',(-2.05725127278289,-0.107036617744751,
28.1016547661024));
#23052=CARTESIAN_POINT('Ctrl Pts',(-2.05634566411282,-0.00160712594267667,
28.0959252805377));
#23053=CARTESIAN_POINT('Ctrl Pts',(-2.05269153525815,-0.00250469671298928,
28.8540747194623));
#23054=CARTESIAN_POINT('Ctrl Pts',(-2.04912674980779,0.46771732011864,28.8286277343138));
#23055=CARTESIAN_POINT('Ctrl Pts',(-1.65657263400563,1.62959319222768,28.7661363765015));
#23056=CARTESIAN_POINT('Ctrl Pts',(0.271806531570387,2.41264813750898,28.6666006460253));
#23057=CARTESIAN_POINT('Ctrl Pts',(2.17449559304179,1.08136903079269,28.5554675280338));
#23058=CARTESIAN_POINT('Ctrl Pts',(2.08783197155072,-1.24094928383581,28.4443344100422));
#23059=CARTESIAN_POINT('Ctrl Pts',(0.0898704340492965,-2.42681281153263,
28.3332012920506));
#23060=CARTESIAN_POINT('Ctrl Pts',(-1.72098255593206,-1.52582831451086,
28.2364480618574));
#23061=CARTESIAN_POINT('Ctrl Pts',(-2.0498856468959,-0.418119100088083,
28.1767392043279));
#23062=CARTESIAN_POINT('Ctrl Pts',(-2.05206134370476,0.00116288414692349,
28.1540747194623));
#23063=CARTESIAN_POINT('Ctrl Pts',(1.26907087985237,1.07935865304853,29.));
#23064=CARTESIAN_POINT('Ctrl Pts',(1.62796789828802,0.657380514756762,28.9629556273361));
#23065=CARTESIAN_POINT('Ctrl Pts',(1.8855124744847,-0.565459156385445,28.8888668820085));
#23066=CARTESIAN_POINT('Ctrl Pts',(0.545109031726074,-1.89347865825101,
28.7777337640169));
#23067=CARTESIAN_POINT('Ctrl Pts',(-1.29391589325212,-1.48358117411062,
28.6666006460253));
#23068=CARTESIAN_POINT('Ctrl Pts',(-1.94881484284809,0.281688560316987,
28.5554675280338));
#23069=CARTESIAN_POINT('Ctrl Pts',(-0.820024337198962,1.7904138164507,28.4443344100422));
#23070=CARTESIAN_POINT('Ctrl Pts',(1.05925521829386,1.65982360610024,28.3332012920507));
#23071=CARTESIAN_POINT('Ctrl Pts',(1.96907801049602,0.0104397431756257,
28.2220681740591));
#23072=CARTESIAN_POINT('Ctrl Pts',(1.07671514955171,-1.64867697221169,28.1109350560675));
#23073=CARTESIAN_POINT('Ctrl Pts',(-0.801095657935827,-1.79876705956693,
27.999801938076));
#23074=CARTESIAN_POINT('Ctrl Pts',(-1.94571434032061,-0.302602882372122,
27.8886688200844));
#23075=CARTESIAN_POINT('Ctrl Pts',(-1.30953755668062,1.47054040479727,27.7775357020928));
#23076=CARTESIAN_POINT('Ctrl Pts',(0.525178959628771,1.89777420920873,27.6664025841013));
#23077=CARTESIAN_POINT('Ctrl Pts',(1.87923132399858,0.588097135770716,27.5552694661097));
#23078=CARTESIAN_POINT('Ctrl Pts',(1.51333705735544,-1.25983310685661,27.4441363481182));
#23079=CARTESIAN_POINT('Ctrl Pts',(-0.237622766646598,-1.95471267106851,
27.3330032301266));
#23080=CARTESIAN_POINT('Ctrl Pts',(-1.771100924469,-0.860563215060856,27.2218701121351));
#23081=CARTESIAN_POINT('Ctrl Pts',(-1.68359778420962,1.02120806251476,27.1107369941435));
#23082=CARTESIAN_POINT('Ctrl Pts',(-0.0551996976013584,1.96832926909851,
26.9996038761519));
#23083=CARTESIAN_POINT('Ctrl Pts',(1.6237193308837,1.11395819001279,26.8884707581604));
#23084=CARTESIAN_POINT('Ctrl Pts',(1.81654651565683,-0.759951339283385,
26.7773376401688));
#23085=CARTESIAN_POINT('Ctrl Pts',(0.346798832347918,-1.93832345519995,
26.6662045221773));
#23086=CARTESIAN_POINT('Ctrl Pts',(-1.44035279303805,-1.34266567211626,
26.5550714041857));
#23087=CARTESIAN_POINT('Ctrl Pts',(-1.90923685006354,0.481852590706729,
26.4439382861942));
#23088=CARTESIAN_POINT('Ctrl Pts',(-0.630712195308838,1.86536039187814,
26.3328051682025));
#23089=CARTESIAN_POINT('Ctrl Pts',(1.22506508530125,1.54161694518754,26.2216720502111));
#23090=CARTESIAN_POINT('Ctrl Pts',(1.95961458169004,-0.193075008570971,
26.1105389322195));
#23091=CARTESIAN_POINT('Ctrl Pts',(0.900647683269863,-1.75105711440899,
25.9994058142279));
#23092=CARTESIAN_POINT('Ctrl Pts',(-0.982627424042958,-1.70640282857695,
25.8882726962363));
#23093=CARTESIAN_POINT('Ctrl Pts',(-1.96656323702446,-0.0999815104761928,
25.7771395782448));
#23094=CARTESIAN_POINT('Ctrl Pts',(-1.15062297231094,1.59794682114526,25.6660064602532));
#23095=CARTESIAN_POINT('Ctrl Pts',(0.718412724742773,1.83337132753311,25.5548733422617));
#23096=CARTESIAN_POINT('Ctrl Pts',(1.92992881966137,0.390822234143067,25.4437402242701));
#23097=CARTESIAN_POINT('Ctrl Pts',(1.3750980975684,-1.40942275053374,25.3326071062786));
#23098=CARTESIAN_POINT('Ctrl Pts',(-0.438276526753214,-1.91970855959058,
25.221473988287));
#23099=CARTESIAN_POINT('Ctrl Pts',(-1.85052322339412,-0.673001535913663,
25.1103408702954));
#23100=CARTESIAN_POINT('Ctrl Pts',(-1.5690982301005,1.18966298251176,24.9992077523039));
#23101=CARTESIAN_POINT('Ctrl Pts',(0.148427222485663,1.96350111466476,24.8880746343123));
#23102=CARTESIAN_POINT('Ctrl Pts',(1.73010623901437,0.940265744025244,24.7769415163208));
#23103=CARTESIAN_POINT('Ctrl Pts',(1.72832392927915,-0.943537844044948,
24.6658083983292));
#23104=CARTESIAN_POINT('Ctrl Pts',(0.144711533300673,-1.96377845995769,
24.5546752803376));
#23105=CARTESIAN_POINT('Ctrl Pts',(-1.57134655374502,-1.1866917357501,24.4435421623461));
#23106=CARTESIAN_POINT('Ctrl Pts',(-1.8492464272056,0.676501972747513,24.3324090443545));
#23107=CARTESIAN_POINT('Ctrl Pts',(-0.434643184857508,1.92053444892845,
24.221275926363));
#23108=CARTESIAN_POINT('Ctrl Pts',(1.37776260766122,1.40681820595075,24.1101428083714));
#23109=CARTESIAN_POINT('Ctrl Pts',(1.9291858334406,-0.394473430938072,23.9990096903799));
#23110=CARTESIAN_POINT('Ctrl Pts',(0.714942252440661,-1.83472745750944,
23.8878765723883));
#23111=CARTESIAN_POINT('Ctrl Pts',(-1.15364461784582,-1.59576670079913,
23.7767434543968));
#23112=CARTESIAN_POINT('Ctrl Pts',(-1.96637052687012,0.103702549247829,
23.6656103364051));
#23113=CARTESIAN_POINT('Ctrl Pts',(-0.979396734113147,1.70825914453061,
23.5544772184136));
#23114=CARTESIAN_POINT('Ctrl Pts',(0.903959498383989,1.74934973431425,23.443344100422));
#23115=CARTESIAN_POINT('Ctrl Pts',(1.95997641846095,0.189366593518892,23.3322109824305));
#23116=CARTESIAN_POINT('Ctrl Pts',(1.22214577644235,-1.54393230706145,23.2210778644389));
#23117=CARTESIAN_POINT('Ctrl Pts',(-0.634240783365302,-1.86416359163571,
23.1099447464473));
#23118=CARTESIAN_POINT('Ctrl Pts',(-1.91014521476306,-0.478238984380987,
22.9988116284558));
#23119=CARTESIAN_POINT('Ctrl Pts',(-1.43780956302664,1.34538876468221,22.8876785104642));
#23120=CARTESIAN_POINT('Ctrl Pts',(0.350465992424694,1.93766376232249,22.7765453924727));
#23121=CARTESIAN_POINT('Ctrl Pts',(1.8179812774019,0.756512618982733,22.6654122744811));
#23122=CARTESIAN_POINT('Ctrl Pts',(1.6216085422551,-1.11702864929655,22.5542791564896));
#23123=CARTESIAN_POINT('Ctrl Pts',(-0.0589241566538478,-1.96822133192042,
22.443146038498));
#23124=CARTESIAN_POINT('Ctrl Pts',(-1.68552714816096,-1.01802038313401,
22.3320129205065));
#23125=CARTESIAN_POINT('Ctrl Pts',(-1.76946935196913,0.863912889188492,
22.2208798025149));
#23126=CARTESIAN_POINT('Ctrl Pts',(-0.233923559220051,1.95515908204568,
22.1097466845233));
#23127=CARTESIAN_POINT('Ctrl Pts',(1.51571828206865,1.25696672870313,21.9986135665318));
#23128=CARTESIAN_POINT('Ctrl Pts',(1.87811509351815,-0.591651048476953,
21.8874804485402));
#23129=CARTESIAN_POINT('Ctrl Pts',(0.521587049489592,-1.89876649893241,
21.7763473305487));
#23130=CARTESIAN_POINT('Ctrl Pts',(-1.31231799169707,-1.46805611484414,
21.6652142125571));
#23131=CARTESIAN_POINT('Ctrl Pts',(-1.94513795455165,0.306277007675757,
21.5540810945656));
#23132=CARTESIAN_POINT('Ctrl Pts',(-0.797691101513079,1.80029335782399,
21.442947976574));
#23133=CARTESIAN_POINT('Ctrl Pts',(1.07983404443909,1.64661036803806,21.3318148585824));
#23134=CARTESIAN_POINT('Ctrl Pts',(1.9690525710802,-0.0141152405335317,
21.2206817405909));
#23135=CARTESIAN_POINT('Ctrl Pts',(1.05611668348891,-1.66192202538936,21.1095486225993));
#23136=CARTESIAN_POINT('Ctrl Pts',(-0.823418761129365,-1.78867236001269,
20.9984155046078));
#23137=CARTESIAN_POINT('Ctrl Pts',(-1.9493289462109,-0.278359349261021,
20.8872823866162));
#23138=CARTESIAN_POINT('Ctrl Pts',(-1.29113655469699,1.48671909398746,20.7761492686246));
#23139=CARTESIAN_POINT('Ctrl Pts',(0.548754829962253,1.89109370584855,20.6650161506331));
#23140=CARTESIAN_POINT('Ctrl Pts',(1.886404196139,0.564664925157129,20.5538830326415));
#23141=CARTESIAN_POINT('Ctrl Pts',(1.49754219255897,-1.27856741957737,20.4427499146499));
#23142=CARTESIAN_POINT('Ctrl Pts',(-0.261929365828814,-1.9516045388674,
20.3316167966584));
#23143=CARTESIAN_POINT('Ctrl Pts',(-1.78167286399379,-0.838456368095613,
20.2204836786668));
#23144=CARTESIAN_POINT('Ctrl Pts',(-1.67075922179782,1.04208006884005,20.1093505606753));
#23145=CARTESIAN_POINT('Ctrl Pts',(-0.0307009971998217,1.96886381712767,
19.9982174426837));
#23146=CARTESIAN_POINT('Ctrl Pts',(1.6374560226953,1.09366589428439,19.8870843246922));
#23147=CARTESIAN_POINT('Ctrl Pts',(1.80694877506856,-0.782498078261772,
19.7759512067006));
#23148=CARTESIAN_POINT('Ctrl Pts',(0.322651014412248,-1.94248905501149,
19.664818088709));
#23149=CARTESIAN_POINT('Ctrl Pts',(-1.45694989770362,-1.32463750790632,
19.5536849707175));
#23150=CARTESIAN_POINT('Ctrl Pts',(-1.90309244999285,0.505574260069482,
19.4425518527259));
#23151=CARTESIAN_POINT('Ctrl Pts',(-0.607450787755709,1.87306488055063,
19.3314187347344));
#23152=CARTESIAN_POINT('Ctrl Pts',(1.24415547621381,1.52625219449683,19.2202856167428));
#23153=CARTESIAN_POINT('Ctrl Pts',(1.95705834927573,-0.217445409941707,
19.1091524987512));
#23154=CARTESIAN_POINT('Ctrl Pts',(0.878790793752254,-1.76213065216931,
18.9980193807597));
#23155=CARTESIAN_POINT('Ctrl Pts',(-1.00379299356237,-1.69404026652977,
18.8868862627681));
#23156=CARTESIAN_POINT('Ctrl Pts',(-1.96764225901355,-0.075505816270981,
18.7757531447766));
#23157=CARTESIAN_POINT('Ctrl Pts',(-1.13067338405636,1.61215041809436,18.664620026785));
#23158=CARTESIAN_POINT('Ctrl Pts',(0.741219758348873,1.8242725863998,18.5534869087934));
#23159=CARTESIAN_POINT('Ctrl Pts',(1.93455119820066,0.366807418669223,18.4423537908019));
#23160=CARTESIAN_POINT('Ctrl Pts',(1.3576286714496,-1.42648727235616,18.3312206728103));
#23161=CARTESIAN_POINT('Ctrl Pts',(-0.462471169546211,-1.91398750101902,
18.2200875548188));
#23162=CARTESIAN_POINT('Ctrl Pts',(-1.85810063661255,-0.650148800818648,
18.1089544368272));
#23163=CARTESIAN_POINT('Ctrl Pts',(-1.55545024827346,1.20953702335538,17.9978213188357));
#23164=CARTESIAN_POINT('Ctrl Pts',(0.175492742231552,1.96063858127948,17.8866882008441));
#23165=CARTESIAN_POINT('Ctrl Pts',(1.21513400202243,1.26723240811114,17.8125994555164));
#23166=CARTESIAN_POINT('Ctrl Pts',(1.47357822736256,0.777253631604911,17.7755550828525));
#23167=CARTESIAN_POINT('Ctrl Pts',(1.36778062465881,1.16331236980976,29.0748149723825));
#23168=CARTESIAN_POINT('Ctrl Pts',(1.75459305244158,0.708512302494195,29.0377705997186));
#23169=CARTESIAN_POINT('Ctrl Pts',(2.032169732279,-0.609441198611308,28.9636818543909));
#23170=CARTESIAN_POINT('Ctrl Pts',(0.587508218617532,-2.0407555346806,28.8525487363994));
#23171=CARTESIAN_POINT('Ctrl Pts',(-1.39455811083951,-1.59897576823537,
28.7414156184078));
#23172=CARTESIAN_POINT('Ctrl Pts',(-2.1003958292741,0.303598609901467,28.6302825004162));
#23173=CARTESIAN_POINT('Ctrl Pts',(-0.883806742378252,1.92967419483109,
28.5191493824247));
#23174=CARTESIAN_POINT('Ctrl Pts',(1.14164526753591,1.78892653264515,28.4080162644331));
#23175=CARTESIAN_POINT('Ctrl Pts',(2.12223508864335,0.0112517580134664,
28.2968831464416));
#23176=CARTESIAN_POINT('Ctrl Pts',(1.1604632516702,-1.77691290117273,28.18575002845));
#23177=CARTESIAN_POINT('Ctrl Pts',(-0.863405769384917,-1.93867716248943,
28.0746169104585));
#23178=CARTESIAN_POINT('Ctrl Pts',(-2.09705416621089,-0.326139671192082,
27.9634837924668));
#23179=CARTESIAN_POINT('Ctrl Pts',(-1.41139484462771,1.58492067337769,27.8523506744754));
#23180=CARTESIAN_POINT('Ctrl Pts',(0.566027963341392,2.04538519837037,27.7412175564837));
#23181=CARTESIAN_POINT('Ctrl Pts',(2.02540002692064,0.633839985216669,27.6300844384923));
#23182=CARTESIAN_POINT('Ctrl Pts',(1.63104609718075,-1.35782432740293,27.5189513205007));
#23183=CARTESIAN_POINT('Ctrl Pts',(-0.256105329778625,-2.10675239713451,
27.4078182025091));
#23184=CARTESIAN_POINT('Ctrl Pts',(-1.90885912462653,-0.92749877925752,
27.2966850845175));
#23185=CARTESIAN_POINT('Ctrl Pts',(-1.81454989277534,1.10063876165494,27.185551966526));
#23186=CARTESIAN_POINT('Ctrl Pts',(-0.059493191487418,2.121428109307,27.0744188485344));
#23187=CARTESIAN_POINT('Ctrl Pts',(1.75001402673825,1.20060309724918,26.9632857305429));
#23188=CARTESIAN_POINT('Ctrl Pts',(1.95783952445267,-0.8190611998569,26.8521526125513));
#23189=CARTESIAN_POINT('Ctrl Pts',(0.373773231322559,-2.08908840982359,
26.7410194945597));
#23190=CARTESIAN_POINT('Ctrl Pts',(-1.55238503559378,-1.44709970173515,
26.6298863765682));
#23191=CARTESIAN_POINT('Ctrl Pts',(-2.05773941618243,0.519331621246395,
26.5187532585766));
#23192=CARTESIAN_POINT('Ctrl Pts',(-0.679769691492573,2.01045019826922,
26.4076201405851));
#23193=CARTESIAN_POINT('Ctrl Pts',(1.32035201045348,1.66152562614826,26.2964870225936));
#23194=CARTESIAN_POINT('Ctrl Pts',(2.11203558381729,-0.208092597522944,
26.1853539046019));
#23195=CARTESIAN_POINT('Ctrl Pts',(0.970701061995584,-1.88725628472242,
26.0742207866104));
#23196=CARTESIAN_POINT('Ctrl Pts',(-1.05905727820396,-1.83912873886292,
25.9630876686188));
#23197=CARTESIAN_POINT('Ctrl Pts',(-2.11952471329362,-0.10775818358496,
25.8519545506273));
#23198=CARTESIAN_POINT('Ctrl Pts',(-1.24011970710203,1.72223690252185,25.7408214326357));
#23199=CARTESIAN_POINT('Ctrl Pts',(0.774291665667894,1.97597298891337,25.6296883146442));
#23200=CARTESIAN_POINT('Ctrl Pts',(2.08004083019426,0.421220822282945,25.5185551966526));
#23201=CARTESIAN_POINT('Ctrl Pts',(1.48205475731824,-1.51904921997551,25.407422078661));
#23202=CARTESIAN_POINT('Ctrl Pts',(-0.4723661625626,-2.06902562692568,25.2962889606695));
#23203=CARTESIAN_POINT('Ctrl Pts',(-1.99445897831498,-0.725348344054207,
25.1851558426779));
#23204=CARTESIAN_POINT('Ctrl Pts',(-1.69114443597316,1.28219629272614,25.0740227246863));
#23205=CARTESIAN_POINT('Ctrl Pts',(0.159972056967716,2.11622441565034,24.9628896066948));
#23206=CARTESIAN_POINT('Ctrl Pts',(1.86467582693291,1.01340065958943,24.8517564887032));
#23207=CARTESIAN_POINT('Ctrl Pts',(1.86275488716375,-1.0169272671887,24.7406233707117));
#23208=CARTESIAN_POINT('Ctrl Pts',(0.155967357344418,-2.11652333316869,
24.6294902527201));
#23209=CARTESIAN_POINT('Ctrl Pts',(-1.69356763673189,-1.27899393908601,
24.5183571347286));
#23210=CARTESIAN_POINT('Ctrl Pts',(-1.99308287149855,0.729121048759038,
24.407224016737));
#23211=CARTESIAN_POINT('Ctrl Pts',(-0.468450215292354,2.06991575485501,
24.2960908987455));
#23212=CARTESIAN_POINT('Ctrl Pts',(1.48492651597021,1.51624209101745,24.1849577807538));
#23213=CARTESIAN_POINT('Ctrl Pts',(2.0792400536787,-0.425156013226423,24.0738246627624));
#23214=CARTESIAN_POINT('Ctrl Pts',(0.770551256169416,-1.97743460018787,
23.9626915447708));
#23215=CARTESIAN_POINT('Ctrl Pts',(-1.24337637958803,-1.71988720998994,
23.8515584267792));
#23216=CARTESIAN_POINT('Ctrl Pts',(-2.11931701392909,0.111768648891705,
23.7404253087876));
#23217=CARTESIAN_POINT('Ctrl Pts',(-1.05557530161745,1.84112944113651,23.6292921907961));
#23218=CARTESIAN_POINT('Ctrl Pts',(0.9742704737735,1.88541610270454,23.5181590728045));
#23219=CARTESIAN_POINT('Ctrl Pts',(2.11242556465477,0.204095737822706,23.407025954813));
#23220=CARTESIAN_POINT('Ctrl Pts',(1.31720563450397,-1.66402107944443,23.2958928368214));
#23221=CARTESIAN_POINT('Ctrl Pts',(-0.68357273705343,-2.00916030957256,
23.1847597188299));
#23222=CARTESIAN_POINT('Ctrl Pts',(-2.05871843449878,-0.515436944600698,
23.0736266008383));
#23223=CARTESIAN_POINT('Ctrl Pts',(-1.54964399032288,1.45003459947016,22.9624934828467));
#23224=CARTESIAN_POINT('Ctrl Pts',(0.377725627189618,2.08837740530025,22.8513603648552));
#23225=CARTESIAN_POINT('Ctrl Pts',(1.95938588356236,0.81535501206587,22.7402272468636));
#23226=CARTESIAN_POINT('Ctrl Pts',(1.74773905862198,-1.20391238027174,22.6290941288721));
#23227=CARTESIAN_POINT('Ctrl Pts',(-0.0635073431082646,-2.12131177665513,
22.5179610108805));
#23228=CARTESIAN_POINT('Ctrl Pts',(-1.81662932480114,-1.09720314102583,
22.406827892889));
#23229=CARTESIAN_POINT('Ctrl Pts',(-1.90710064660258,0.931108994765127,
22.2956947748974));
#23230=CARTESIAN_POINT('Ctrl Pts',(-0.252118393883275,2.1072335304541,22.1845616569058));
#23231=CARTESIAN_POINT('Ctrl Pts',(1.63361253620114,1.35473499916799,22.0734285389142));
#23232=CARTESIAN_POINT('Ctrl Pts',(2.0241969747917,-0.63767032520673,21.9622954209227));
#23233=CARTESIAN_POINT('Ctrl Pts',(0.562156670435786,-2.04645466949263,
21.8511623029311));
#23234=CARTESIAN_POINT('Ctrl Pts',(-1.41439154497283,-1.58224315258837,
21.7400291849396));
#23235=CARTESIAN_POINT('Ctrl Pts',(-2.09643294851562,0.330099574049098,
21.628896066948));
#23236=CARTESIAN_POINT('Ctrl Pts',(-0.859736402776227,1.94032217792285,
21.5177629489565));
#23237=CARTESIAN_POINT('Ctrl Pts',(1.16382473767152,1.7746855542275,21.4066298309649));
#23238=CARTESIAN_POINT('Ctrl Pts',(2.12220767052146,-0.0152131396446604,
21.2954967129734));
#23239=CARTESIAN_POINT('Ctrl Pts',(1.13826261400238,-1.79118816932096,21.1843635949818));
#23240=CARTESIAN_POINT('Ctrl Pts',(-0.887465188378072,-1.92779728597407,
21.0732304769903));
#23241=CARTESIAN_POINT('Ctrl Pts',(-2.10094992016838,-0.300010449106,20.9620973589987));
#23242=CARTESIAN_POINT('Ctrl Pts',(-1.3915625922397,1.60235775901099,20.8509642410071));
#23243=CARTESIAN_POINT('Ctrl Pts',(0.591437591096275,2.03818507802715,20.7398311230155));
#23244=CARTESIAN_POINT('Ctrl Pts',(2.03313081303557,0.608585191194508,20.628698005024));
#23245=CARTESIAN_POINT('Ctrl Pts',(1.6140226902295,-1.378015815808,20.5175648870324));
#23246=CARTESIAN_POINT('Ctrl Pts',(-0.282302523284989,-2.10340251095318,
20.4064317690409));
#23247=CARTESIAN_POINT('Ctrl Pts',(-1.92025336136826,-0.903672437142665,
20.2952986510493));
#23248=CARTESIAN_POINT('Ctrl Pts',(-1.80071273269696,1.12313421585117,20.1841655330578));
#23249=CARTESIAN_POINT('Ctrl Pts',(-0.0330889549151928,2.12200423507653,
20.0730324150662));
#23250=CARTESIAN_POINT('Ctrl Pts',(1.76481917372027,1.17873244418496,19.9618992970747));
#23251=CARTESIAN_POINT('Ctrl Pts',(1.94749526092448,-0.843361649275031,
19.8507661790831));
#23252=CARTESIAN_POINT('Ctrl Pts',(0.347747169244733,-2.09357801462248,
19.7396330610915));
#23253=CARTESIAN_POINT('Ctrl Pts',(-1.5702730815236,-1.42766928685762,19.6284999431));
#23254=CARTESIAN_POINT('Ctrl Pts',(-2.05111709783893,0.544898388441233,
19.5173668251084));
#23255=CARTESIAN_POINT('Ctrl Pts',(-0.654698985782925,2.01875395064148,
19.4062337071168));
#23256=CARTESIAN_POINT('Ctrl Pts',(1.34092727320823,1.64496578805638,19.2951005891253));
#23257=CARTESIAN_POINT('Ctrl Pts',(2.10928052480214,-0.234358555823027,
19.1839674711337));
#23258=CARTESIAN_POINT('Ctrl Pts',(0.947144119296707,-1.89919113456843,
19.0728343531422));
#23259=CARTESIAN_POINT('Ctrl Pts',(-1.08186912926612,-1.82580460298704,
18.9617012351506));
#23260=CARTESIAN_POINT('Ctrl Pts',(-2.12068766281338,-0.0813787426566056,
18.8505681171591));
#23261=CARTESIAN_POINT('Ctrl Pts',(-1.21861841768019,1.73754527104238,18.7394349991675));
#23262=CARTESIAN_POINT('Ctrl Pts',(0.798872655719443,1.96616653757285,18.6283018811759));
#23263=CARTESIAN_POINT('Ctrl Pts',(2.08502274247847,0.395338107746388,18.5171687631844));
#23264=CARTESIAN_POINT('Ctrl Pts',(1.46322653980215,-1.53744103928863,18.4060356451928));
#23265=CARTESIAN_POINT('Ctrl Pts',(-0.498442691587246,-2.06285957805406,
18.2949025272013));
#23266=CARTESIAN_POINT('Ctrl Pts',(-2.00262577116299,-0.700718097801093,
18.1837694092097));
#23267=CARTESIAN_POINT('Ctrl Pts',(-1.67643489893699,1.30361615857535,18.0726362912181));
#23268=CARTESIAN_POINT('Ctrl Pts',(0.189142762948342,2.11313923123394,17.9615031732266));
#23269=CARTESIAN_POINT('Ctrl Pts',(1.30964847646945,1.36579915454035,17.8874144278989));
#23270=CARTESIAN_POINT('Ctrl Pts',(1.58819478116152,0.83770928372304,17.850370055235));
#23271=CARTESIAN_POINT('Ctrl Pts',(1.46649036946526,1.24726608657098,29.149629944765));
#23272=CARTESIAN_POINT('Ctrl Pts',(1.88121820659513,0.759644090231628,29.1125855721011));
#23273=CARTESIAN_POINT('Ctrl Pts',(2.1788269900733,-0.653423240837164,29.0384968267735));
#23274=CARTESIAN_POINT('Ctrl Pts',(0.629907405508992,-2.18803241111019,
28.9273637087818));
#23275=CARTESIAN_POINT('Ctrl Pts',(-1.49520032842689,-1.71437036236012,
28.8162305907904));
#23276=CARTESIAN_POINT('Ctrl Pts',(-2.25197681570011,0.325508659485947,
28.7050974727987));
#23277=CARTESIAN_POINT('Ctrl Pts',(-0.947589147557543,2.06893457321149,
28.5939643548072));
#23278=CARTESIAN_POINT('Ctrl Pts',(1.22403531677795,1.91802945919006,28.4828312368156));
#23279=CARTESIAN_POINT('Ctrl Pts',(2.27539216679067,0.0120637728513067,
28.3716981188241));
#23280=CARTESIAN_POINT('Ctrl Pts',(1.2442113537887,-1.90514883013378,28.2605650008325));
#23281=CARTESIAN_POINT('Ctrl Pts',(-0.925715880834006,-2.07858726541193,
28.1494318828409));
#23282=CARTESIAN_POINT('Ctrl Pts',(-2.24839399210117,-0.349676460012044,
28.0382987648494));
#23283=CARTESIAN_POINT('Ctrl Pts',(-1.51325213257481,1.69930094195811,27.9271656468578));
#23284=CARTESIAN_POINT('Ctrl Pts',(0.606876967054013,2.19299618753202,27.8160325288663));
#23285=CARTESIAN_POINT('Ctrl Pts',(2.1715687298427,0.67958283466262,27.7048994108747));
#23286=CARTESIAN_POINT('Ctrl Pts',(1.74875513700607,-1.45581554794925,27.5937662928831));
#23287=CARTESIAN_POINT('Ctrl Pts',(-0.274587892910651,-2.25879212320052,
27.4826331748916));
#23288=CARTESIAN_POINT('Ctrl Pts',(-2.04661732478405,-0.994434343454176,
27.3715000569));
#23289=CARTESIAN_POINT('Ctrl Pts',(-1.94550200134107,1.18006946079512,27.2603669389085));
#23290=CARTESIAN_POINT('Ctrl Pts',(-0.0637866853734778,2.27452694951549,
27.1492338209169));
#23291=CARTESIAN_POINT('Ctrl Pts',(1.8763087225928,1.28724800448557,27.0381007029253));
#23292=CARTESIAN_POINT('Ctrl Pts',(2.09913253324851,-0.878171060430411,
26.9269675849338));
#23293=CARTESIAN_POINT('Ctrl Pts',(0.400747630297199,-2.23985336444724,
26.8158344669422));
#23294=CARTESIAN_POINT('Ctrl Pts',(-1.66441727814951,-1.55153373135404,
26.7047013489507));
#23295=CARTESIAN_POINT('Ctrl Pts',(-2.20624198230131,0.556810651786059,
26.5935682309591));
#23296=CARTESIAN_POINT('Ctrl Pts',(-0.728827187676307,2.1555400046603,26.4824351129675));
#23297=CARTESIAN_POINT('Ctrl Pts',(1.41563893560571,1.78143430710897,26.371301994976));
#23298=CARTESIAN_POINT('Ctrl Pts',(2.26445658594454,-0.223110186474918,
26.2601688769844));
#23299=CARTESIAN_POINT('Ctrl Pts',(1.04075444072131,-2.02345545503584,26.1490357589928));
#23300=CARTESIAN_POINT('Ctrl Pts',(-1.13548713236497,-1.97185464914889,
26.0379026410014));
#23301=CARTESIAN_POINT('Ctrl Pts',(-2.27248618956277,-0.115534856693729,
25.9267695230097));
#23302=CARTESIAN_POINT('Ctrl Pts',(-1.32961644189312,1.84652698389845,25.8156364050182));
#23303=CARTESIAN_POINT('Ctrl Pts',(0.830170606593015,2.11857465029362,25.7045032870266));
#23304=CARTESIAN_POINT('Ctrl Pts',(2.23015284072714,0.451619410422826,25.5933701690351));
#23305=CARTESIAN_POINT('Ctrl Pts',(1.58901141706808,-1.62867568941729,25.4822370510435));
#23306=CARTESIAN_POINT('Ctrl Pts',(-0.506455798371986,-2.21834269426078,
25.371103933052));
#23307=CARTESIAN_POINT('Ctrl Pts',(-2.13839473323584,-0.777695152194749,
25.2599708150604));
#23308=CARTESIAN_POINT('Ctrl Pts',(-1.81319064184582,1.37472960294051,25.1488376970688));
#23309=CARTESIAN_POINT('Ctrl Pts',(0.17151689144977,2.26894771663592,25.0377045790773));
#23310=CARTESIAN_POINT('Ctrl Pts',(1.99924541485144,1.08653557515362,24.9265714610857));
#23311=CARTESIAN_POINT('Ctrl Pts',(1.99718584504836,-1.09031669033245,24.8154383430942));
#23312=CARTESIAN_POINT('Ctrl Pts',(0.167223181388163,-2.26926820637968,
24.7043052251026));
#23313=CARTESIAN_POINT('Ctrl Pts',(-1.81578871971876,-1.37129614242191,
24.5931721071111));
#23314=CARTESIAN_POINT('Ctrl Pts',(-2.13691931579151,0.781740124770563,
24.4820389891195));
#23315=CARTESIAN_POINT('Ctrl Pts',(-0.502257245727199,2.21929706078156,
24.370905871128));
#23316=CARTESIAN_POINT('Ctrl Pts',(1.59209042427919,1.62566597608415,24.2597727531364));
#23317=CARTESIAN_POINT('Ctrl Pts',(2.22929427391681,-0.455838595514776,
24.1486396351449));
#23318=CARTESIAN_POINT('Ctrl Pts',(0.826160259898167,-2.1201417428663,24.0375065171532));
#23319=CARTESIAN_POINT('Ctrl Pts',(-1.33310814133023,-1.84400771918075,
23.9263733991618));
#23320=CARTESIAN_POINT('Ctrl Pts',(-2.27226350098807,0.119834748535584,
23.8152402811701));
#23321=CARTESIAN_POINT('Ctrl Pts',(-1.13175386912174,1.97399973774241,23.7041071631786));
#23322=CARTESIAN_POINT('Ctrl Pts',(1.04458144916301,2.02148247109483,23.592974045187));
#23323=CARTESIAN_POINT('Ctrl Pts',(2.26487471084858,0.218824882126523,23.4818409271955));
#23324=CARTESIAN_POINT('Ctrl Pts',(1.41226549256559,-1.78410985182741,23.3707078092039));
#23325=CARTESIAN_POINT('Ctrl Pts',(-0.732904690741557,-2.15415702750941,
23.2595746912124));
#23326=CARTESIAN_POINT('Ctrl Pts',(-2.2072916542345,-0.552634904820408,
23.1484415732208));
#23327=CARTESIAN_POINT('Ctrl Pts',(-1.66147841761912,1.55468043425812,23.0373084552292));
#23328=CARTESIAN_POINT('Ctrl Pts',(0.404985261954545,2.23909104827802,22.9261753372377));
#23329=CARTESIAN_POINT('Ctrl Pts',(2.10079048972282,0.874197405149011,22.8150422192461));
#23330=CARTESIAN_POINT('Ctrl Pts',(1.87386957498886,-1.29079611124694,22.7039091012546));
#23331=CARTESIAN_POINT('Ctrl Pts',(-0.0680905295626852,-2.27440222138984,
22.592775983263));
#23332=CARTESIAN_POINT('Ctrl Pts',(-1.9477315014413,-1.17638589891765,22.4816428652714));
#23333=CARTESIAN_POINT('Ctrl Pts',(-2.04473194123603,0.998305100341762,
22.3705097472799));
#23334=CARTESIAN_POINT('Ctrl Pts',(-0.270313228546498,2.25930797886252,
22.2593766292883));
#23335=CARTESIAN_POINT('Ctrl Pts',(1.75150679033363,1.45250326963284,22.1482435112967));
#23336=CARTESIAN_POINT('Ctrl Pts',(2.17027885606524,-0.683689601936504,
22.0371103933052));
#23337=CARTESIAN_POINT('Ctrl Pts',(0.60272629138198,-2.19414284005285,21.9259772753136));
#23338=CARTESIAN_POINT('Ctrl Pts',(-1.51646509824859,-1.6964301903326,21.8148441573221));
#23339=CARTESIAN_POINT('Ctrl Pts',(-2.2477279424796,0.353922140422439,21.7037110393305));
#23340=CARTESIAN_POINT('Ctrl Pts',(-0.921781704039374,2.0803509980217,21.592577921339));
#23341=CARTESIAN_POINT('Ctrl Pts',(1.24781543090395,1.90276074041694,21.4814448033474));
#23342=CARTESIAN_POINT('Ctrl Pts',(2.27536276996272,-0.0163110387557863,
21.3703116853558));
#23343=CARTESIAN_POINT('Ctrl Pts',(1.22040854451584,-1.92045431325255,21.2591785673643));
#23344=CARTESIAN_POINT('Ctrl Pts',(-0.951511615626781,-2.06692221193544,
21.1480454493727));
#23345=CARTESIAN_POINT('Ctrl Pts',(-2.25257089412586,-0.321661548950983,
21.0369123313812));
#23346=CARTESIAN_POINT('Ctrl Pts',(-1.49198862978241,1.71799642403453,20.9257792133896));
#23347=CARTESIAN_POINT('Ctrl Pts',(0.634120352230293,2.18527645020575,20.814646095398));
#23348=CARTESIAN_POINT('Ctrl Pts',(2.17985742993213,0.652505457231891,20.7035129774065));
#23349=CARTESIAN_POINT('Ctrl Pts',(1.73050318790003,-1.47746421203863,20.5923798594149));
#23350=CARTESIAN_POINT('Ctrl Pts',(-0.302675680741162,-2.25520048303895,
20.4812467414234));
#23351=CARTESIAN_POINT('Ctrl Pts',(-2.05883385874272,-0.968888506189718,
20.3701136234318));
#23352=CARTESIAN_POINT('Ctrl Pts',(-1.9306662435961,1.20418836286229,20.2589805054403));
#23353=CARTESIAN_POINT('Ctrl Pts',(-0.0354769126305643,2.27514465302538,
20.1478473874487));
#23354=CARTESIAN_POINT('Ctrl Pts',(1.89218232474523,1.26379899408554,20.0367142694571));
#23355=CARTESIAN_POINT('Ctrl Pts',(2.0880417467804,-0.904225220288291,19.9255811514656));
#23356=CARTESIAN_POINT('Ctrl Pts',(0.372843324077218,-2.24466697423347,
19.814448033474));
#23357=CARTESIAN_POINT('Ctrl Pts',(-1.68359626534358,-1.53070106580892,
19.7033149154824));
#23358=CARTESIAN_POINT('Ctrl Pts',(-2.19914174568501,0.584222516812984,
19.5921817974909));
#23359=CARTESIAN_POINT('Ctrl Pts',(-0.701947183810143,2.16444302073233,
19.4810486794993));
#23360=CARTESIAN_POINT('Ctrl Pts',(1.43769907020265,1.76367938161593,19.3699155615078));
#23361=CARTESIAN_POINT('Ctrl Pts',(2.26150270032853,-0.251271701704347,
19.2587824435162));
#23362=CARTESIAN_POINT('Ctrl Pts',(1.01549744484116,-2.03625161696756,19.1476493255247));
#23363=CARTESIAN_POINT('Ctrl Pts',(-1.15994526496988,-1.95756893944432,
19.0365162075331));
#23364=CARTESIAN_POINT('Ctrl Pts',(-2.2737330666132,-0.087251669042228,
18.9253830895416));
#23365=CARTESIAN_POINT('Ctrl Pts',(-1.30656345130402,1.86294012399039,18.81424997155));
#23366=CARTESIAN_POINT('Ctrl Pts',(0.856525553090016,2.1080604887459,18.7031168535584));
#23367=CARTESIAN_POINT('Ctrl Pts',(2.23549428675628,0.423868796823551,18.5919837355669));
#23368=CARTESIAN_POINT('Ctrl Pts',(1.5688244081547,-1.6483948062211,18.4808506175753));
#23369=CARTESIAN_POINT('Ctrl Pts',(-0.53441421362828,-2.2117316550891,18.3697174995838));
#23370=CARTESIAN_POINT('Ctrl Pts',(-2.14715090571344,-0.751287394783537,
18.2585843815922));
#23371=CARTESIAN_POINT('Ctrl Pts',(-1.79741954960052,1.39769529379532,18.1474512636006));
#23372=CARTESIAN_POINT('Ctrl Pts',(0.202792783665131,2.2656398811884,18.0363181456091));
#23373=CARTESIAN_POINT('Ctrl Pts',(1.40416295091648,1.46436590096956,17.9622294002814));
#23374=CARTESIAN_POINT('Ctrl Pts',(1.70281133496047,0.898164935841169,17.9251850276175));
#23375=CARTESIAN_POINT('Ctrl Pts',(1.5652001142717,1.33121980333221,29.2244449171475));
#23376=CARTESIAN_POINT('Ctrl Pts',(2.00784336074869,0.810775877969061,29.1874005444836));
#23377=CARTESIAN_POINT('Ctrl Pts',(2.32548424786761,-0.697405283063022,
29.1133117991559));
#23378=CARTESIAN_POINT('Ctrl Pts',(0.67230659240045,-2.33530928753977,29.0021786811644));
#23379=CARTESIAN_POINT('Ctrl Pts',(-1.59584254601428,-1.82976495648487,
28.8910455631728));
#23380=CARTESIAN_POINT('Ctrl Pts',(-2.40355780212611,0.347418709070426,
28.7799124451812));
#23381=CARTESIAN_POINT('Ctrl Pts',(-1.01137155273683,2.20819495159188,28.6687793271897));
#23382=CARTESIAN_POINT('Ctrl Pts',(1.30642536602,2.04713238573498,28.5576462091981));
#23383=CARTESIAN_POINT('Ctrl Pts',(2.428549244938,0.0128757876891458,28.4465130912066));
#23384=CARTESIAN_POINT('Ctrl Pts',(1.32795945590719,-2.03338475909482,28.335379973215));
#23385=CARTESIAN_POINT('Ctrl Pts',(-0.988025992283097,-2.21849736833443,
28.2242468552234));
#23386=CARTESIAN_POINT('Ctrl Pts',(-2.39973381799145,-0.373213248832005,
28.1131137372319));
#23387=CARTESIAN_POINT('Ctrl Pts',(-1.61510942052191,1.81368121053853,28.0019806192403));
#23388=CARTESIAN_POINT('Ctrl Pts',(0.647725970766636,2.34060717669366,27.8908475012488));
#23389=CARTESIAN_POINT('Ctrl Pts',(2.31773743276476,0.725325684108574,27.7797143832572));
#23390=CARTESIAN_POINT('Ctrl Pts',(1.86646417683138,-1.55380676849557,27.6685812652656));
#23391=CARTESIAN_POINT('Ctrl Pts',(-0.293070456042677,-2.41083184926652,
27.5574481472741));
#23392=CARTESIAN_POINT('Ctrl Pts',(-2.18437552494158,-1.06136990765084,
27.4463150292825));
#23393=CARTESIAN_POINT('Ctrl Pts',(-2.07645410990679,1.2595001599353,27.335181911291));
#23394=CARTESIAN_POINT('Ctrl Pts',(-0.0680801792595378,2.42762578972398,
27.2240487932994));
#23395=CARTESIAN_POINT('Ctrl Pts',(2.00260341844735,1.37389291172196,27.1129156753079));
#23396=CARTESIAN_POINT('Ctrl Pts',(2.24042554204435,-0.937280921003925,
27.0017825573163));
#23397=CARTESIAN_POINT('Ctrl Pts',(0.427722029271838,-2.39061831907088,
26.8906494393248));
#23398=CARTESIAN_POINT('Ctrl Pts',(-1.77644952070524,-1.65596776097293,
26.7795163213331));
#23399=CARTESIAN_POINT('Ctrl Pts',(-2.3547445484202,0.594289682325723,26.6683832033416));
#23400=CARTESIAN_POINT('Ctrl Pts',(-0.777884683860044,2.30062981105139,
26.5572500853501));
#23401=CARTESIAN_POINT('Ctrl Pts',(1.51092586075795,1.90134298806969,26.4461169673585));
#23402=CARTESIAN_POINT('Ctrl Pts',(2.4168775880718,-0.238127775426892,26.3349838493669));
#23403=CARTESIAN_POINT('Ctrl Pts',(1.11080781944703,-2.15965462534927,26.2238507313753));
#23404=CARTESIAN_POINT('Ctrl Pts',(-1.21191698652597,-2.10458055943487,
26.1127176133838));
#23405=CARTESIAN_POINT('Ctrl Pts',(-2.42544766583193,-0.123311529802495,
26.0015844953922));
#23406=CARTESIAN_POINT('Ctrl Pts',(-1.41911317668421,1.97081706527504,25.8904513774007));
#23407=CARTESIAN_POINT('Ctrl Pts',(0.886049547518136,2.26117631167387,25.7793182594091));
#23408=CARTESIAN_POINT('Ctrl Pts',(2.38026485126002,0.482017998562706,25.6681851414176));
#23409=CARTESIAN_POINT('Ctrl Pts',(1.69596807681793,-1.73830215885906,25.557052023426));
#23410=CARTESIAN_POINT('Ctrl Pts',(-0.540545434181373,-2.36765976159588,
25.4459189054345));
#23411=CARTESIAN_POINT('Ctrl Pts',(-2.2823304881567,-0.830041960335293,
25.3347857874429));
#23412=CARTESIAN_POINT('Ctrl Pts',(-1.93523684771849,1.46726291315489,25.2236526694514));
#23413=CARTESIAN_POINT('Ctrl Pts',(0.183061725931824,2.4216710176215,25.1125195514598));
#23414=CARTESIAN_POINT('Ctrl Pts',(2.13381500276998,1.15967049071781,25.0013864334682));
#23415=CARTESIAN_POINT('Ctrl Pts',(2.13161680293297,-1.1637061134762,24.8902533154767));
#23416=CARTESIAN_POINT('Ctrl Pts',(0.178479005431905,-2.42201307959068,
24.7791201974851));
#23417=CARTESIAN_POINT('Ctrl Pts',(-1.93800980270562,-1.46359834575782,
24.6679870794936));
#23418=CARTESIAN_POINT('Ctrl Pts',(-2.28075576008446,0.834359200782086,
24.556853961502));
#23419=CARTESIAN_POINT('Ctrl Pts',(-0.536064276162042,2.36867836670812,
24.4457208435105));
#23420=CARTESIAN_POINT('Ctrl Pts',(1.69925433258817,1.73508986115085,24.3345877255189));
#23421=CARTESIAN_POINT('Ctrl Pts',(2.37934849415491,-0.486521177803125,
24.2234546075274));
#23422=CARTESIAN_POINT('Ctrl Pts',(0.881769263626921,-2.26284888554473,
24.1123214895357));
#23423=CARTESIAN_POINT('Ctrl Pts',(-1.42283990307244,-1.96812822837156,
24.0011883715443));
#23424=CARTESIAN_POINT('Ctrl Pts',(-2.42520998804704,0.127900848179458,
23.8900552535526));
#23425=CARTESIAN_POINT('Ctrl Pts',(-1.20793243662604,2.10687003434831,23.7789221355611));
#23426=CARTESIAN_POINT('Ctrl Pts',(1.11489242455252,2.15754883948512,23.6677890175695));
#23427=CARTESIAN_POINT('Ctrl Pts',(2.4173238570424,0.233554026430338,23.556655899578));
#23428=CARTESIAN_POINT('Ctrl Pts',(1.50732535062721,-1.90419862421039,23.4455227815864));
#23429=CARTESIAN_POINT('Ctrl Pts',(-0.782236644429685,-2.29915374544626,
23.3343896635949));
#23430=CARTESIAN_POINT('Ctrl Pts',(-2.35586487397022,-0.589832865040116,
23.2232565456033));
#23431=CARTESIAN_POINT('Ctrl Pts',(-1.77331284491536,1.65932626904607,23.1121234276117));
#23432=CARTESIAN_POINT('Ctrl Pts',(0.43224489671947,2.38980469125578,23.0009903096202));
#23433=CARTESIAN_POINT('Ctrl Pts',(2.24219509588329,0.933039798232153,22.8898571916286));
#23434=CARTESIAN_POINT('Ctrl Pts',(2.00000009135574,-1.37767984222214,22.778724073637));
#23435=CARTESIAN_POINT('Ctrl Pts',(-0.072673716017103,-2.42749266612454,
22.6675909556455));
#23436=CARTESIAN_POINT('Ctrl Pts',(-2.07883367808147,-1.25556865680948,
22.5564578376539));
#23437=CARTESIAN_POINT('Ctrl Pts',(-2.18236323586949,1.0655012059184,22.4453247196624));
#23438=CARTESIAN_POINT('Ctrl Pts',(-0.288508063209722,2.41138242727093,
22.3341916016708));
#23439=CARTESIAN_POINT('Ctrl Pts',(1.86940104446612,1.5502715400977,22.2230584836792));
#23440=CARTESIAN_POINT('Ctrl Pts',(2.31636073733878,-0.729708878666279,
22.1119253656877));
#23441=CARTESIAN_POINT('Ctrl Pts',(0.643295912328174,-2.34183101061307,
22.0007922476961));
#23442=CARTESIAN_POINT('Ctrl Pts',(-1.61853865152434,-1.81061722807683,
21.8896591297046));
#23443=CARTESIAN_POINT('Ctrl Pts',(-2.39902293644358,0.377744706795778,
21.778526011713));
#23444=CARTESIAN_POINT('Ctrl Pts',(-0.983827005302519,2.22037981812055,
21.6673928937214));
#23445=CARTESIAN_POINT('Ctrl Pts',(1.33180612413638,2.03083592660637,21.5562597757299));
#23446=CARTESIAN_POINT('Ctrl Pts',(2.42851786940399,-0.0174089378669135,
21.4451266577383));
#23447=CARTESIAN_POINT('Ctrl Pts',(1.30255447502931,-2.04972045718415,21.3339935397468));
#23448=CARTESIAN_POINT('Ctrl Pts',(-1.01555804287549,-2.20604713789681,
21.2228604217552));
#23449=CARTESIAN_POINT('Ctrl Pts',(-2.40419186808334,-0.343312648795965,
21.1117273037636));
#23450=CARTESIAN_POINT('Ctrl Pts',(-1.59241466732511,1.83363508905806,21.0005941857721));
#23451=CARTESIAN_POINT('Ctrl Pts',(0.676803113364313,2.33236782238435,20.8894610677805));
#23452=CARTESIAN_POINT('Ctrl Pts',(2.3265840468287,0.696425723269271,20.778327949789));
#23453=CARTESIAN_POINT('Ctrl Pts',(1.84698368557056,-1.57691260826926,20.6671948317974));
#23454=CARTESIAN_POINT('Ctrl Pts',(-0.323048838197336,-2.40699845512473,
20.5560617138059));
#23455=CARTESIAN_POINT('Ctrl Pts',(-2.19741435611719,-1.03410457523677,
20.4449285958143));
#23456=CARTESIAN_POINT('Ctrl Pts',(-2.06061975449524,1.2852425098734,20.3337954778227));
#23457=CARTESIAN_POINT('Ctrl Pts',(-0.037864870345937,2.42828507097424,
20.2226623598312));
#23458=CARTESIAN_POINT('Ctrl Pts',(2.01954547577021,1.34886554398611,20.1115292418396));
#23459=CARTESIAN_POINT('Ctrl Pts',(2.22858823263633,-0.965088791301547,
20.0003961238481));
#23460=CARTESIAN_POINT('Ctrl Pts',(0.397939478909703,-2.39575593384446,
19.8892630058565));
#23461=CARTESIAN_POINT('Ctrl Pts',(-1.79691944916357,-1.63373284476021,
19.7781298878649));
#23462=CARTESIAN_POINT('Ctrl Pts',(-2.34716639353109,0.623546645184736,
19.6669967698734));
#23463=CARTESIAN_POINT('Ctrl Pts',(-0.74919538183736,2.31013209082318,19.5558636518818));
#23464=CARTESIAN_POINT('Ctrl Pts',(1.53447086719707,1.88239297517548,19.4447305338903));
#23465=CARTESIAN_POINT('Ctrl Pts',(2.41372487585493,-0.268184847585669,
19.3335974158987));
#23466=CARTESIAN_POINT('Ctrl Pts',(1.08385077038562,-2.17331209936668,19.2224642979071));
#23467=CARTESIAN_POINT('Ctrl Pts',(-1.23802140067364,-2.08933327590159,
19.1113311799156));
#23468=CARTESIAN_POINT('Ctrl Pts',(-2.42677847041303,-0.0931245954278493,
19.000198061924));
#23469=CARTESIAN_POINT('Ctrl Pts',(-1.39450848492785,1.98833497693841,18.8890649439325));
#23470=CARTESIAN_POINT('Ctrl Pts',(0.91417845046059,2.24995443991895,18.7779318259409));
#23471=CARTESIAN_POINT('Ctrl Pts',(2.38596583103409,0.452399485900713,18.6667987079494));
#23472=CARTESIAN_POINT('Ctrl Pts',(1.67442227650725,-1.75934857315356,18.5556655899578));
#23473=CARTESIAN_POINT('Ctrl Pts',(-0.570385735669315,-2.36060373212415,
18.4445324719663));
#23474=CARTESIAN_POINT('Ctrl Pts',(-2.29167604026388,-0.801856691765977,
18.3333993539747));
#23475=CARTESIAN_POINT('Ctrl Pts',(-1.91840420026404,1.49177442901529,18.2222662359831));
#23476=CARTESIAN_POINT('Ctrl Pts',(0.216442804381921,2.41814053114287,18.1111331179916));
#23477=CARTESIAN_POINT('Ctrl Pts',(1.4986774253635,1.56293264739877,18.0370443726639));
#23478=CARTESIAN_POINT('Ctrl Pts',(1.81742788875943,0.958620587959298,18.));
#23479=CARTESIAN_POINT('Ctrl Pts',(1.26907087985237,1.07935865304853,29.));
#23480=CARTESIAN_POINT('Ctrl Pts',(1.3144094872273,1.03706254429827,29.));
#23481=CARTESIAN_POINT('Ctrl Pts',(1.35701863562271,0.992198004702034,29.));
#23482=CARTESIAN_POINT('Ctrl Pts',(1.39689941920223,0.945109875853942,29.));
#23483=CARTESIAN_POINT('Ctrl Pts',(1.43940262027365,0.894925400302773,29.));
#23484=CARTESIAN_POINT('Ctrl Pts',(1.47880756852856,0.842215055268869,29.));
#23485=CARTESIAN_POINT('Ctrl Pts',(1.51508678956216,0.787341601735945,29.));
#23486=CARTESIAN_POINT('Ctrl Pts',(1.54683110796656,0.739327329894636,29.));
#23487=CARTESIAN_POINT('Ctrl Pts',(1.57618204898653,0.689655703631122,29.));
#23488=CARTESIAN_POINT('Ctrl Pts',(1.60309832979504,0.638542209490663,29.));
#23489=CARTESIAN_POINT('Ctrl Pts',(1.61660467751284,0.612893917668903,29.));
#23490=CARTESIAN_POINT('Ctrl Pts',(1.62949763128333,0.586882216194757,29.));
#23491=CARTESIAN_POINT('Ctrl Pts',(1.64176963246512,0.560532489670278,29.));
#23492=CARTESIAN_POINT('Ctrl Pts',(1.64737448368887,0.548498079408378,29.));
#23493=CARTESIAN_POINT('Ctrl Pts',(1.65285037736292,0.536391499107776,29.));
#23494=CARTESIAN_POINT('Ctrl Pts',(1.65818810198435,0.524235070687702,29.));
#23495=CARTESIAN_POINT('Ctrl Pts',(1.68511823217932,0.462902907026757,29.));
#23496=CARTESIAN_POINT('Ctrl Pts',(1.70858664543798,0.400195370245674,29.));
#23497=CARTESIAN_POINT('Ctrl Pts',(1.72856940504418,0.336469942157596,29.));
#23498=CARTESIAN_POINT('Ctrl Pts',(1.7489050278493,0.271619226128731,29.));
#23499=CARTESIAN_POINT('Ctrl Pts',(1.76563136617229,0.205713511440919,29.));
#23500=CARTESIAN_POINT('Ctrl Pts',(1.77868388077386,0.139093051206905,29.));
#23501=CARTESIAN_POINT('Ctrl Pts',(1.7895994088527,0.0833798398826602,29.));
#23502=CARTESIAN_POINT('Ctrl Pts',(1.79794505461674,0.0271658230940875,
29.));
#23503=CARTESIAN_POINT('Ctrl Pts',(1.80365825317042,-0.0293622786831205,
29.));
#23504=CARTESIAN_POINT('Ctrl Pts',(1.80629075136643,-0.0554090061956506,
29.));
#23505=CARTESIAN_POINT('Ctrl Pts',(1.80836401037494,-0.0815225313140194,
29.));
#23506=CARTESIAN_POINT('Ctrl Pts',(1.8098701058109,-0.107684989121531,29.));
#23507=CARTESIAN_POINT('Ctrl Pts',(1.81052758192083,-0.119106038926533,
29.));
#23508=CARTESIAN_POINT('Ctrl Pts',(1.81107685493986,-0.130536175706242,
29.));
#23509=CARTESIAN_POINT('Ctrl Pts',(1.81151693302746,-0.141959838006402,
29.));
#23510=CARTESIAN_POINT('Ctrl Pts',(1.81421811506976,-0.212077829181081,
29.));
#23511=CARTESIAN_POINT('Ctrl Pts',(1.81281756748119,-0.282083201198475,
29.));
#23512=CARTESIAN_POINT('Ctrl Pts',(1.80726021940794,-0.351615623243351,
29.));
#23513=CARTESIAN_POINT('Ctrl Pts',(1.80229344163224,-0.413758948432297,
29.));
#23514=CARTESIAN_POINT('Ctrl Pts',(1.79400604326908,-0.475525464431958,
29.));
#23515=CARTESIAN_POINT('Ctrl Pts',(1.78232561606514,-0.536670064275249,
29.));
#23516=CARTESIAN_POINT('Ctrl Pts',(1.76959660145245,-0.603303800465088,
29.));
#23517=CARTESIAN_POINT('Ctrl Pts',(1.75283909722983,-0.669199777224924,
29.));
#23518=CARTESIAN_POINT('Ctrl Pts',(1.73229861749773,-0.734144131843436,
29.));
#23519=CARTESIAN_POINT('Ctrl Pts',(1.72436741483446,-0.759220802156505,
29.));
#23520=CARTESIAN_POINT('Ctrl Pts',(1.71587164297147,-0.784155545451161,
29.));
#23521=CARTESIAN_POINT('Ctrl Pts',(1.70682342442655,-0.808935730194906,
29.));
#23522=CARTESIAN_POINT('Ctrl Pts',(1.70285503775051,-0.819803875618098,
29.));
#23523=CARTESIAN_POINT('Ctrl Pts',(1.6987804849517,-0.830641729526751,29.));
#23524=CARTESIAN_POINT('Ctrl Pts',(1.69460587821655,-0.841435680151886,
29.));
#23525=CARTESIAN_POINT('Ctrl Pts',(1.6693812505011,-0.906657005984914,29.));
#23526=CARTESIAN_POINT('Ctrl Pts',(1.64046524049148,-0.970394630379315,
29.));
#23527=CARTESIAN_POINT('Ctrl Pts',(1.60817079267237,-1.03242943870664,29.));
#23528=CARTESIAN_POINT('Ctrl Pts',(1.57512648034544,-1.09590467113643,29.));
#23529=CARTESIAN_POINT('Ctrl Pts',(1.53854471445853,-1.15759791168999,29.));
#23530=CARTESIAN_POINT('Ctrl Pts',(1.49870459830356,-1.21727074006036,29.));
#23531=CARTESIAN_POINT('Ctrl Pts',(1.46819625766185,-1.26296636423716,29.));
#23532=CARTESIAN_POINT('Ctrl Pts',(1.43577599564766,-1.30747724665079,29.));
#23533=CARTESIAN_POINT('Ctrl Pts',(1.40154956798818,-1.35069022138389,29.));
#23534=CARTESIAN_POINT('Ctrl Pts',(1.38024570649905,-1.37758765974371,29.));
#23535=CARTESIAN_POINT('Ctrl Pts',(1.35824175768608,-1.40398212651681,29.));
#23536=CARTESIAN_POINT('Ctrl Pts',(1.33556031487129,-1.42984464135766,29.));
#23537=CARTESIAN_POINT('Ctrl Pts',(1.32288534609529,-1.44429727432079,29.));
#23538=CARTESIAN_POINT('Ctrl Pts',(1.3099943443598,-1.45858831293731,29.));
#23539=CARTESIAN_POINT('Ctrl Pts',(1.29691491924979,-1.47268731356655,29.));
#23540=CARTESIAN_POINT('Ctrl Pts',(1.24603363784778,-1.52753492441104,29.));
#23541=CARTESIAN_POINT('Ctrl Pts',(1.19225580967216,-1.57953769268553,29.));
#23542=CARTESIAN_POINT('Ctrl Pts',(1.1358667874795,-1.62843129863239,29.));
#23543=CARTESIAN_POINT('Ctrl Pts',(1.09369930723698,-1.6649937372522,29.));
#23544=CARTESIAN_POINT('Ctrl Pts',(1.05007049363608,-1.69981733826376,29.));
#23545=CARTESIAN_POINT('Ctrl Pts',(1.00508328076865,-1.73278182943765,29.));
#23546=CARTESIAN_POINT('Ctrl Pts',(0.991019284017403,-1.74308725774107,
29.));
#23547=CARTESIAN_POINT('Ctrl Pts',(0.976822434853456,-1.75321091355829,
29.));
#23548=CARTESIAN_POINT('Ctrl Pts',(0.962495636971034,-1.76314889540177,
29.));
#23549=CARTESIAN_POINT('Ctrl Pts',(0.948702692966066,-1.77271656210681,
29.));
#23550=CARTESIAN_POINT('Ctrl Pts',(0.934796339602229,-1.78210719109177,
29.));
#23551=CARTESIAN_POINT('Ctrl Pts',(0.920784555255717,-1.79131455083345,
29.));
#23552=CARTESIAN_POINT('Ctrl Pts',(0.857822233634552,-1.83268806408493,
29.));
#23553=CARTESIAN_POINT('Ctrl Pts',(0.792703365228481,-1.87038503190709,
29.));
#23554=CARTESIAN_POINT('Ctrl Pts',(0.725689641419005,-1.90412588607056,
29.));
#23555=CARTESIAN_POINT('Ctrl Pts',(0.674455559543145,-1.92992182138804,
29.));
#23556=CARTESIAN_POINT('Ctrl Pts',(0.622112945371267,-1.95340496957484,
29.));
#23557=CARTESIAN_POINT('Ctrl Pts',(0.568764876142657,-1.97443513991583,
29.));
#23558=CARTESIAN_POINT('Ctrl Pts',(0.556316873757165,-1.97934222679559,
29.));
#23559=CARTESIAN_POINT('Ctrl Pts',(0.543814084655739,-1.98411569285989,
29.));
#23560=CARTESIAN_POINT('Ctrl Pts',(0.531258445741635,-1.98875612844697,
29.));
#23561=CARTESIAN_POINT('Ctrl Pts',(-1.66729377121886,-0.00130306451899955,
27.8714803633902));
#23562=CARTESIAN_POINT('Ctrl Pts',(-1.66802804256299,-0.0867857428702756,
27.8772098489549));
#23563=CARTESIAN_POINT('Ctrl Pts',(-1.66202149744119,-0.172164864355061,
27.8829393345197));
#23564=CARTESIAN_POINT('Ctrl Pts',(-1.64891509598314,-0.256439697376359,
27.8886688200844));
#23565=CARTESIAN_POINT('Ctrl Pts',(-1.56417477952568,-0.801324274770393,
27.9257131927483));
#23566=CARTESIAN_POINT('Ctrl Pts',(-1.18263521873075,-1.30004566716866,
27.9627575654121));
#23567=CARTESIAN_POINT('Ctrl Pts',(-0.678896970418698,-1.52439134880859,
27.999801938076));
#23568=CARTESIAN_POINT('Ctrl Pts',(-0.175158722106646,-1.74873703044852,
28.0368463107398));
#23569=CARTESIAN_POINT('Ctrl Pts',(0.450778213722533,-1.69870700133011,
28.0738906834037));
#23570=CARTESIAN_POINT('Ctrl Pts',(0.912473825127841,-1.39717253420635,
28.1109350560675));
#23571=CARTESIAN_POINT('Ctrl Pts',(1.37416943653315,-1.09563806708259,28.1479794287314));
#23572=CARTESIAN_POINT('Ctrl Pts',(1.67162372351458,-0.542599161953481,
28.1850238013952));
#23573=CARTESIAN_POINT('Ctrl Pts',(1.66871373497161,0.0088176010985061,
28.2220681740591));
#23574=CARTESIAN_POINT('Ctrl Pts',(1.66580374642864,0.560234364150496,28.2591125467229));
#23575=CARTESIAN_POINT('Ctrl Pts',(1.36252948236125,1.11002898512537,28.2961569193868));
#23576=CARTESIAN_POINT('Ctrl Pts',(0.897679091078753,1.40669133067121,28.3332012920506));
#23577=CARTESIAN_POINT('Ctrl Pts',(0.432828699796255,1.70335367621706,28.3702456647145));
#23578=CARTESIAN_POINT('Ctrl Pts',(-0.193597818701355,1.74688374633388,
28.4072900373784));
#23579=CARTESIAN_POINT('Ctrl Pts',(-0.69494282889168,1.51719457203667,28.4443344100422));
#23580=CARTESIAN_POINT('Ctrl Pts',(-1.196287839082,1.28750539773946,28.4813787827061));
#23581=CARTESIAN_POINT('Ctrl Pts',(-1.57255134096505,0.784596979028224,
28.5184231553699));
#23582=CARTESIAN_POINT('Ctrl Pts',(-1.65153326697391,0.238931147268006,
28.5554675280338));
#23583=CARTESIAN_POINT('Ctrl Pts',(-1.66291353417212,0.160307805445838,
28.5608051398193));
#23584=CARTESIAN_POINT('Ctrl Pts',(-1.66812192138366,0.0807967744989645,
28.5661427516047));
#23585=CARTESIAN_POINT('Ctrl Pts',(-1.66745735078673,0.00120170187390745,
28.5714803633902));
#23586=CARTESIAN_POINT('Ctrl Pts',(-0.530170217188634,-1.98517432567172,
29.));
#23587=CARTESIAN_POINT('Ctrl Pts',(-1.19025956241812,-1.80888768575368,
28.9629556273361));
#23588=CARTESIAN_POINT('Ctrl Pts',(-2.30934991790679,-0.749104679977639,
28.8888668820084));
#23589=CARTESIAN_POINT('Ctrl Pts',(-1.88125738141003,1.53835568783795,28.7777337640169));
#23590=CARTESIAN_POINT('Ctrl Pts',(0.271806531570387,2.41264813750898,28.6666006460253));
#23591=CARTESIAN_POINT('Ctrl Pts',(2.17449559304179,1.08136903079269,28.5554675280338));
#23592=CARTESIAN_POINT('Ctrl Pts',(2.08783197155072,-1.24094928383581,28.4443344100422));
#23593=CARTESIAN_POINT('Ctrl Pts',(0.0898704340492965,-2.42681281153263,
28.3332012920506));
#23594=CARTESIAN_POINT('Ctrl Pts',(-1.99011943914583,-1.39192006204976,
28.2220681740591));
#23595=CARTESIAN_POINT('Ctrl Pts',(-2.24879050981126,0.917099090480224,
28.1109350560675));
#23596=CARTESIAN_POINT('Ctrl Pts',(-0.449219217968869,2.38665611117453,
27.999801938076));
#23597=CARTESIAN_POINT('Ctrl Pts',(1.76146356868064,1.6719019509933,27.8886688200844));
#23598=CARTESIAN_POINT('Ctrl Pts',(2.36000201199169,-0.573068912759941,
27.7775357020928));
#23599=CARTESIAN_POINT('Ctrl Pts',(0.798565170672349,-2.29353090612058,
27.6664025841013));
#23600=CARTESIAN_POINT('Ctrl Pts',(-1.49374549619868,-1.91487023989728,
27.5552694661097));
#23601=CARTESIAN_POINT('Ctrl Pts',(-2.4189238064285,0.216358730773912,27.4441363481182));
#23602=CARTESIAN_POINT('Ctrl Pts',(-1.13020663702663,2.14956575456656,27.3330032301266));
#23603=CARTESIAN_POINT('Ctrl Pts',(1.19291950474651,2.1154065927935,27.2218701121351));
#23604=CARTESIAN_POINT('Ctrl Pts',(2.42423908872827,0.145143535993706,27.1107369941435));
#23605=CARTESIAN_POINT('Ctrl Pts',(1.43679947210715,-1.95796032739892,26.999603876152));
#23606=CARTESIAN_POINT('Ctrl Pts',(-0.865655485103571,-2.26906197521519,
26.8884707581604));
#23607=CARTESIAN_POINT('Ctrl Pts',(-2.37582851633814,-0.503428720754339,
26.7773376401688));
#23608=CARTESIAN_POINT('Ctrl Pts',(-1.71154975386622,1.72296227565052,26.6662045221772));
#23609=CARTESIAN_POINT('Ctrl Pts',(0.51920669687721,2.37243040203942,26.5550714041857));
#23610=CARTESIAN_POINT('Ctrl Pts',(2.27476474931693,0.850556836234861,26.4439382861941));
#23611=CARTESIAN_POINT('Ctrl Pts',(1.9483685659561,-1.44977981832677,26.3328051682026));
#23612=CARTESIAN_POINT('Ctrl Pts',(-0.161251214260656,-2.42322092316419,
26.221672050211));
#23613=CARTESIAN_POINT('Ctrl Pts',(-2.12328753730864,-1.17883486062637,
26.1105389322195));
#23614=CARTESIAN_POINT('Ctrl Pts',(-2.14200753395606,1.14446726409082,25.9994058142279));
#23615=CARTESIAN_POINT('Ctrl Pts',(-0.200277927177756,2.42030790331167,
25.8882726962363));
#23616=CARTESIAN_POINT('Ctrl Pts',(1.92475392154391,1.48098748682692,25.7771395782448));
#23617=CARTESIAN_POINT('Ctrl Pts',(2.28817522362595,-0.813790968595164,
25.6660064602532));
#23618=CARTESIAN_POINT('Ctrl Pts',(0.557368499380946,-2.36375589911376,
25.5548733422617));
#23619=CARTESIAN_POINT('Ctrl Pts',(-1.68356381332587,-1.75031839420915,
25.4437402242701));
#23620=CARTESIAN_POINT('Ctrl Pts',(-2.38363225964151,0.465079396921421,
25.3326071062785));
#23621=CARTESIAN_POINT('Ctrl Pts',(-0.902106643086596,2.25481821865058,
25.221473988287));
#23622=CARTESIAN_POINT('Ctrl Pts',(1.40506247979517,1.98085865788643,25.1103408702954));
#23623=CARTESIAN_POINT('Ctrl Pts',(2.42626311844678,-0.106060712410309,
24.9992077523039));
#23624=CARTESIAN_POINT('Ctrl Pts',(1.22685225431082,-2.09590914420127,24.8880746343123));
#23625=CARTESIAN_POINT('Ctrl Pts',(-1.09542208140494,-2.16749903303861,
24.7769415163207));
#23626=CARTESIAN_POINT('Ctrl Pts',(-2.41512301282573,-0.255308494908708,
24.6658083983292));
#23627=CARTESIAN_POINT('Ctrl Pts',(-1.52440830459303,1.89055042660624,24.5546752803376));
#23628=CARTESIAN_POINT('Ctrl Pts',(0.761504884129454,2.30610318635139,24.4435421623461));
#23629=CARTESIAN_POINT('Ctrl Pts',(2.35045883035646,0.611019542610869,24.3324090443546));
#23630=CARTESIAN_POINT('Ctrl Pts',(1.7881803418832,-1.64329323602198,24.2212759263629));
#23631=CARTESIAN_POINT('Ctrl Pts',(-0.410711177573986,-2.39359936565602,
24.1101428083714));
#23632=CARTESIAN_POINT('Ctrl Pts',(-2.23370366188104,-0.953189144688686,
23.9990096903798));
#23633=CARTESIAN_POINT('Ctrl Pts',(-2.01232263711515,1.35961729865687,23.8878765723883));
#23634=CARTESIAN_POINT('Ctrl Pts',(0.0508152693856986,2.42804847625626,
23.7767434543967));
#23635=CARTESIAN_POINT('Ctrl Pts',(2.06744504127525,1.27423412132916,23.6656103364052));
#23636=CARTESIAN_POINT('Ctrl Pts',(2.19186773754582,-1.04580945480468,23.5544772184136));
#23637=CARTESIAN_POINT('Ctrl Pts',(0.310206809340991,-2.40868705524225,
23.443344100422));
#23638=CARTESIAN_POINT('Ctrl Pts',(-1.85536760039376,-1.56703945772346,
23.3322109824305));
#23639=CARTESIAN_POINT('Ctrl Pts',(-2.322836555691,0.708824329575872,23.2210778644389));
#23640=CARTESIAN_POINT('Ctrl Pts',(-0.664354069263913,2.33594419139362,
23.1099447464474));
#23641=CARTESIAN_POINT('Ctrl Pts',(1.60217141007485,1.82511598738049,22.9988116284558));
#23642=CARTESIAN_POINT('Ctrl Pts',(2.40232655406092,-0.356130204148507,
22.8876785104642));
#23643=CARTESIAN_POINT('Ctrl Pts',(1.00377788111867,-2.21143201569255,22.7765453924727));
#23644=CARTESIAN_POINT('Ctrl Pts',(-1.3134678169358,-2.04274420535881,22.6654122744811));
#23645=CARTESIAN_POINT('Ctrl Pts',(-2.42857607134113,-0.00445649665224475,
22.5542791564896));
#23646=CARTESIAN_POINT('Ctrl Pts',(-1.32095591743234,2.03790997319645,22.443146038498));
#23647=CARTESIAN_POINT('Ctrl Pts',(0.995655084428766,2.21510102422083,22.3320129205065));
#23648=CARTESIAN_POINT('Ctrl Pts',(2.40100336441846,0.364944432351608,22.2208798025149));
#23649=CARTESIAN_POINT('Ctrl Pts',(1.60885886272077,-1.81922366807872,22.1097466845233));
#23650=CARTESIAN_POINT('Ctrl Pts',(-0.655776594206566,-2.33836666353754,
21.9986135665318));
#23651=CARTESIAN_POINT('Ctrl Pts',(-2.32021950100116,-0.717344451311874,
21.8874804485402));
#23652=CARTESIAN_POINT('Ctrl Pts',(-1.86110619752919,1.56021963715706,21.7763473305487));
#23653=CARTESIAN_POINT('Ctrl Pts',(0.301364750346359,2.40980930405301,21.6652142125571));
#23654=CARTESIAN_POINT('Ctrl Pts',(2.18801481710634,1.05384664671037,21.5540810945656));
#23655=CARTESIAN_POINT('Ctrl Pts',(2.07210760382199,-1.2666379407027,21.442947976574));
#23656=CARTESIAN_POINT('Ctrl Pts',(0.0597259541680415,-2.42784563039867,
21.3318148585825));
#23657=CARTESIAN_POINT('Ctrl Pts',(-2.00731923954813,-1.36699344008564,
21.2206817405908));
#23658=CARTESIAN_POINT('Ctrl Pts',(-2.23718685788182,0.944984950940279,
21.1095486225994));
#23659=CARTESIAN_POINT('Ctrl Pts',(-0.419493009128206,2.39207592060309,
20.9984155046077));
#23660=CARTESIAN_POINT('Ctrl Pts',(1.7821373527842,1.64984485657254,20.8872823866162));
#23661=CARTESIAN_POINT('Ctrl Pts',(2.35268546495377,-0.602389157518069,
20.7761492686246));
#23662=CARTESIAN_POINT('Ctrl Pts',(0.769963239246222,-2.30329290471873,
20.6650161506331));
#23663=CARTESIAN_POINT('Ctrl Pts',(-1.51745964933489,-1.89613232903235,
20.5538830326415));
#23664=CARTESIAN_POINT('Ctrl Pts',(-2.41604373856618,0.24644318568101,20.44274991465));
#23665=CARTESIAN_POINT('Ctrl Pts',(-1.10336950687639,2.16346419607446,20.3316167966584));
#23666=CARTESIAN_POINT('Ctrl Pts',(1.21915193180051,2.10039762278245,20.2204836786668));
#23667=CARTESIAN_POINT('Ctrl Pts',(2.42585752542742,0.114964471039976,20.1093505606753));
#23668=CARTESIAN_POINT('Ctrl Pts',(1.41232285348001,-1.97568868333651,19.9982174426837));
#23669=CARTESIAN_POINT('Ctrl Pts',(-0.893825325748239,-2.2581138043306,
19.8870843246922));
#23670=CARTESIAN_POINT('Ctrl Pts',(-2.38190930300825,-0.4738242701237,19.7759512067006));
#23671=CARTESIAN_POINT('Ctrl Pts',(-1.68997629510449,1.74412784145651,19.6648180887091));
#23672=CARTESIAN_POINT('Ctrl Pts',(0.548689842456826,2.36578558927548,19.5536849707175));
#23673=CARTESIAN_POINT('Ctrl Pts',(2.28517284872419,0.82218308608128,19.4425518527259));
#23674=CARTESIAN_POINT('Ctrl Pts',(1.93017685695003,-1.47391342438527,19.3314187347344));
#23675=CARTESIAN_POINT('Ctrl Pts',(-0.191395150412758,-2.42102695967158,
19.2202856167428));
#23676=CARTESIAN_POINT('Ctrl Pts',(-2.13779058223796,-1.15232017062793,
19.1091524987513));
#23677=CARTESIAN_POINT('Ctrl Pts',(-2.12760400594706,1.17103316317459,18.9980193807597));
#23678=CARTESIAN_POINT('Ctrl Pts',(-0.170134977547301,2.42261514214274,
18.8868862627681));
#23679=CARTESIAN_POINT('Ctrl Pts',(1.9430184348445,1.45691614743391,18.7757531447766));
#23680=CARTESIAN_POINT('Ctrl Pts',(2.27790227156009,-0.842194003777161,
18.664620026785));
#23681=CARTESIAN_POINT('Ctrl Pts',(0.52784999826971,-2.37052551568832,18.5534869087934));
#23682=CARTESIAN_POINT('Ctrl Pts',(-1.70509933605923,-1.72920021145774,
18.4423537908019));
#23683=CARTESIAN_POINT('Ctrl Pts',(-2.37788229208364,0.494644591072267,
18.3312206728103));
#23684=CARTESIAN_POINT('Ctrl Pts',(-0.873549834886296,2.26598780907704,
18.2200875548188));
#23685=CARTESIAN_POINT('Ctrl Pts',(1.42878011639417,1.96299190141644,18.1089544368272));
#23686=CARTESIAN_POINT('Ctrl Pts',(2.42636094490168,-0.135794412509918,
17.9978213188357));
#23687=CARTESIAN_POINT('Ctrl Pts',(1.19738788458608,-2.11199363605741,17.8866882008441));
#23688=CARTESIAN_POINT('Ctrl Pts',(-0.343660854083971,-2.13791714127778,
17.8125994555164));
#23689=CARTESIAN_POINT('Ctrl Pts',(-0.949553552261494,-1.82218155349229,
17.7755550828525));
#23690=CARTESIAN_POINT('Ctrl Pts',(-0.496734897087716,-1.85997880000276,
29.0748149723825));
#23691=CARTESIAN_POINT('Ctrl Pts',(-1.11519553923768,-1.69480972203762,
29.0377705997186));
#23692=CARTESIAN_POINT('Ctrl Pts',(-2.16371017575061,-0.70186220208636,
28.9636818543909));
#23693=CARTESIAN_POINT('Ctrl Pts',(-1.76261540436122,1.441338893638,28.8525487363994));
#23694=CARTESIAN_POINT('Ctrl Pts',(0.254664983263946,2.26049386676127,28.7414156184078));
#23695=CARTESIAN_POINT('Ctrl Pts',(2.03736047331189,1.01317221678926,28.6302825004163));
#23696=CARTESIAN_POINT('Ctrl Pts',(1.95616231523563,-1.16268850043293,28.5191493824247));
#23697=CARTESIAN_POINT('Ctrl Pts',(0.0842027321818088,-2.27376524200133,
28.4080162644332));
#23698=CARTESIAN_POINT('Ctrl Pts',(-1.86461204863313,-1.30413826797557,
28.2968831464416));
#23699=CARTESIAN_POINT('Ctrl Pts',(-2.1069699621876,0.859262002201165,28.18575002845));
#23700=CARTESIAN_POINT('Ctrl Pts',(-0.42088909330076,2.23614103420343,28.0746169104585));
#23701=CARTESIAN_POINT('Ctrl Pts',(1.65037641901529,1.56646302761273,27.9634837924669));
#23702=CARTESIAN_POINT('Ctrl Pts',(2.21116788259043,-0.536928175470663,
27.8523506744754));
#23703=CARTESIAN_POINT('Ctrl Pts',(0.748203454308011,-2.14888879398133,
27.7412175564837));
#23704=CARTESIAN_POINT('Ctrl Pts',(-1.39954205512358,-1.79410845934652,
27.6300844384923));
#23705=CARTESIAN_POINT('Ctrl Pts',(-2.26637375901817,0.202714012180677,
27.5189513205007));
#23706=CARTESIAN_POINT('Ctrl Pts',(-1.05892986691768,2.01400284146476,27.4078182025091));
#23707=CARTESIAN_POINT('Ctrl Pts',(1.11768773162403,1.98199793594985,27.2966850845176));
#23708=CARTESIAN_POINT('Ctrl Pts',(2.27135383168271,0.135990021840718,27.185551966526));
#23709=CARTESIAN_POINT('Ctrl Pts',(1.34618734657985,-1.83448105947885,27.0744188485344));
#23710=CARTESIAN_POINT('Ctrl Pts',(-0.811062700931283,-2.12596300245047,
26.9632857305429));
#23711=CARTESIAN_POINT('Ctrl Pts',(-2.22599628439971,-0.47167985995323,
26.8521526125513));
#23712=CARTESIAN_POINT('Ctrl Pts',(-1.60361043167528,1.61430321985961,26.7410194945598));
#23713=CARTESIAN_POINT('Ctrl Pts',(0.486462793983747,2.22281247304678,26.6298863765682));
#23714=CARTESIAN_POINT('Ctrl Pts',(2.13130612964755,0.796916252208208,26.5187532585767));
#23715=CARTESIAN_POINT('Ctrl Pts',(1.82549420492022,-1.35834908395122,26.4076201405851));
#23716=CARTESIAN_POINT('Ctrl Pts',(-0.151081865265427,-2.27039987698986,
26.2964870225935));
#23717=CARTESIAN_POINT('Ctrl Pts',(-1.98938186668712,-1.10449133918118,
26.185353904602));
#23718=CARTESIAN_POINT('Ctrl Pts',(-2.0069212819667,1.07229114389529,26.0742207866104));
#23719=CARTESIAN_POINT('Ctrl Pts',(-0.187647348568785,2.26767056747804,
25.9630876686188));
#23720=CARTESIAN_POINT('Ctrl Pts',(1.80336882408676,1.38758863287,25.8519545506273));
#23721=CARTESIAN_POINT('Ctrl Pts',(2.14387086897055,-0.762469033397635,
25.7408214326357));
#23722=CARTESIAN_POINT('Ctrl Pts',(0.522217912669773,-2.21468502986276,
25.6296883146442));
#23723=CARTESIAN_POINT('Ctrl Pts',(-1.57738943161999,-1.63993411781724,
25.5185551966526));
#23724=CARTESIAN_POINT('Ctrl Pts',(-2.23330788263933,0.435749046018521,
25.407422078661));
#23725=CARTESIAN_POINT('Ctrl Pts',(-0.845215057330029,2.11261753203009,
25.2962889606695));
#23726=CARTESIAN_POINT('Ctrl Pts',(1.31645185579057,1.85593530090815,25.1851558426779));
#23727=CARTESIAN_POINT('Ctrl Pts',(2.27325021545028,-0.0993719665045596,
25.0740227246864));
#23728=CARTESIAN_POINT('Ctrl Pts',(1.14948050367395,-1.96373009893084,24.9628896066948));
#23729=CARTESIAN_POINT('Ctrl Pts',(-1.02633900817686,-2.03080515315156,
24.8517564887032));
#23730=CARTESIAN_POINT('Ctrl Pts',(-2.26281266343432,-0.239207399496329,
24.7406233707117));
#23731=CARTESIAN_POINT('Ctrl Pts',(-1.42827110567824,1.77132238128959,24.6294902527201));
#23732=CARTESIAN_POINT('Ctrl Pts',(0.713480384197537,2.16066820014965,24.5183571347286));
#23733=CARTESIAN_POINT('Ctrl Pts',(2.20222654414142,0.572485439161143,24.407224016737));
#23734=CARTESIAN_POINT('Ctrl Pts',(1.67540829209497,-1.53965852855496,24.2960908987454));
#23735=CARTESIAN_POINT('Ctrl Pts',(-0.384809572304588,-2.24264641056841,
24.1849577807539));
#23736=CARTESIAN_POINT('Ctrl Pts',(-2.09283457017381,-0.893076027927082,
24.0738246627623));
#23737=CARTESIAN_POINT('Ctrl Pts',(-1.88541499625397,1.27387268660304,23.9626915447708));
#23738=CARTESIAN_POINT('Ctrl Pts',(0.0476105914486115,2.2749229792137,23.8515584267792));
#23739=CARTESIAN_POINT('Ctrl Pts',(1.93706109192281,1.19387422115205,23.7404253087876));
#23740=CARTESIAN_POINT('Ctrl Pts',(2.05363703908762,-0.979855214539392,
23.6292921907961));
#23741=CARTESIAN_POINT('Ctrl Pts',(0.290643537713249,-2.25678259115896,
23.5181590728045));
#23742=CARTESIAN_POINT('Ctrl Pts',(-1.73835836899447,-1.46821371425264,
23.407025954813));
#23743=CARTESIAN_POINT('Ctrl Pts',(-2.17634627527977,0.664122142266367,
23.2958928368214));
#23744=CARTESIAN_POINT('Ctrl Pts',(-0.622456410274362,2.18862727459039,
23.1847597188299));
#23745=CARTESIAN_POINT('Ctrl Pts',(1.5011300610597,1.7100145816792,23.0736266008383));
#23746=CARTESIAN_POINT('Ctrl Pts',(2.25082321660849,-0.333670761902858,
22.9624934828467));
#23747=CARTESIAN_POINT('Ctrl Pts',(0.940474372778667,-2.07196749103822,
22.8513603648552));
#23748=CARTESIAN_POINT('Ctrl Pts',(-1.23063363372879,-1.91391802052963,
22.7402272468636));
#23749=CARTESIAN_POINT('Ctrl Pts',(-2.27541730137984,-0.00417544655311686,
22.629094128872));
#23750=CARTESIAN_POINT('Ctrl Pts',(-1.23764949525578,1.90938866045279,22.5179610108805));
#23751=CARTESIAN_POINT('Ctrl Pts',(0.93286384233578,2.07540511260695,22.4068278928889));
#23752=CARTESIAN_POINT('Ctrl Pts',(2.24958347425864,0.341929118554036,22.2956947748974));
#23753=CARTESIAN_POINT('Ctrl Pts',(1.50739576779718,-1.70449386299853,22.1845616569058));
#23754=CARTESIAN_POINT('Ctrl Pts',(-0.614419875871358,-2.1908969729101,
22.0734285389143));
#23755=CARTESIAN_POINT('Ctrl Pts',(-2.1738942658121,-0.672104940349877,
21.9622954209227));
#23756=CARTESIAN_POINT('Ctrl Pts',(-1.74373506003647,1.46182398741138,21.8511623029312));
#23757=CARTESIAN_POINT('Ctrl Pts',(0.282359105426515,2.25783406506196,21.7400291849396));
#23758=CARTESIAN_POINT('Ctrl Pts',(2.05002710405932,0.987385538885627,21.628896066948));
#23759=CARTESIAN_POINT('Ctrl Pts',(1.94142960877218,-1.18675709559613,21.5177629489565));
#23760=CARTESIAN_POINT('Ctrl Pts',(0.0559593216202335,-2.2747329258819,
21.4066298309649));
#23761=CARTESIAN_POINT('Ctrl Pts',(-1.8807271392319,-1.28078364978945,21.2954967129733));
#23762=CARTESIAN_POINT('Ctrl Pts',(-2.09609809752954,0.885389233751969,
21.1843635949818));
#23763=CARTESIAN_POINT('Ctrl Pts',(-0.393037575409816,2.24121904196669,
21.0732304769902));
#23764=CARTESIAN_POINT('Ctrl Pts',(1.66974640564629,1.54579696948286,20.9620973589987));
#23765=CARTESIAN_POINT('Ctrl Pts',(2.20431275545938,-0.564399331507581,
20.8509642410071));
#23766=CARTESIAN_POINT('Ctrl Pts',(0.721405310989425,-2.15803514964562,
20.7398311230156));
#23767=CARTESIAN_POINT('Ctrl Pts',(-1.42176066913796,-1.77655225961412,
20.628698005024));
#23768=CARTESIAN_POINT('Ctrl Pts',(-2.26367532337088,0.230901183258412,
20.5175648870324));
#23769=CARTESIAN_POINT('Ctrl Pts',(-1.03378522723196,2.02702477421066,20.4064317690409));
#23770=CARTESIAN_POINT('Ctrl Pts',(1.14226580396866,1.96793551046437,20.2952986510493));
#23771=CARTESIAN_POINT('Ctrl Pts',(2.27287020125823,0.107714207323098,20.1841655330578));
#23772=CARTESIAN_POINT('Ctrl Pts',(1.32325435215538,-1.85109137212314,20.0730324150662));
#23773=CARTESIAN_POINT('Ctrl Pts',(-0.837456003383859,-2.11570528075782,
19.9618992970746));
#23774=CARTESIAN_POINT('Ctrl Pts',(-2.23169358470602,-0.443942421559709,
19.8507661790831));
#23775=CARTESIAN_POINT('Ctrl Pts',(-1.58339750859812,1.63413397385441,19.7396330610915));
#23776=CARTESIAN_POINT('Ctrl Pts',(0.514086577460258,2.21658671709625,19.6284999431));
#23777=CARTESIAN_POINT('Ctrl Pts',(2.14105783960848,0.770331899851958,19.5173668251084));
#23778=CARTESIAN_POINT('Ctrl Pts',(1.80844976068701,-1.38096069798226,19.4062337071169));
#23779=CARTESIAN_POINT('Ctrl Pts',(-0.179324766388269,-2.26834427636504,
19.2951005891253));
#23780=CARTESIAN_POINT('Ctrl Pts',(-2.00297027338529,-1.07964880487677,
19.1839674711338));
#23781=CARTESIAN_POINT('Ctrl Pts',(-1.99342611612885,1.097181657771,19.0728343531422));
#23782=CARTESIAN_POINT('Ctrl Pts',(-0.159405371752351,2.26983229970319,
18.9617012351506));
#23783=CARTESIAN_POINT('Ctrl Pts',(1.82048148119308,1.36503535864129,18.850568117159));
#23784=CARTESIAN_POINT('Ctrl Pts',(2.13424578324943,-0.789080823914506,
18.7394349991675));
#23785=CARTESIAN_POINT('Ctrl Pts',(0.494561003367273,-2.22102771883975,
18.6283018811759));
#23786=CARTESIAN_POINT('Ctrl Pts',(-1.5975668111141,-1.62014775865258,18.5171687631844));
#23787=CARTESIAN_POINT('Ctrl Pts',(-2.22792053825349,0.463449703652169,
18.4060356451928));
#23788=CARTESIAN_POINT('Ctrl Pts',(-0.818459191529514,2.12308270938467,
18.2949025272012));
#23789=CARTESIAN_POINT('Ctrl Pts',(1.33867373358228,1.83919531599638,18.1837694092097));
#23790=CARTESIAN_POINT('Ctrl Pts',(2.27334187245483,-0.127230503216293,
18.0726362912181));
#23791=CARTESIAN_POINT('Ctrl Pts',(1.12187431194823,-1.97880021820166,17.9615031732266));
#23792=CARTESIAN_POINT('Ctrl Pts',(-0.321987794583605,-2.00308885094696,
17.8874144278989));
#23793=CARTESIAN_POINT('Ctrl Pts',(-0.889669715064486,-1.70726520861333,
17.850370055235));
#23794=CARTESIAN_POINT('Ctrl Pts',(-0.463299576986798,-1.7347832743338,
29.149629944765));
#23795=CARTESIAN_POINT('Ctrl Pts',(-1.04013151605724,-1.58073175832155,
29.1125855721011));
#23796=CARTESIAN_POINT('Ctrl Pts',(-2.01807043359442,-0.654619724195083,
29.0384968267734));
#23797=CARTESIAN_POINT('Ctrl Pts',(-1.64397342731241,1.34432209943806,28.9273637087818));
#23798=CARTESIAN_POINT('Ctrl Pts',(0.237523434957504,2.10833959601355,28.8162305907903));
#23799=CARTESIAN_POINT('Ctrl Pts',(1.900225353582,0.944975402785826,28.7050974727987));
#23800=CARTESIAN_POINT('Ctrl Pts',(1.82449265892053,-1.08442771703006,28.5939643548072));
#23801=CARTESIAN_POINT('Ctrl Pts',(0.0785350303143197,-2.12071767247004,
28.4828312368156));
#23802=CARTESIAN_POINT('Ctrl Pts',(-1.73910465812042,-1.21635647390137,
28.3716981188241));
#23803=CARTESIAN_POINT('Ctrl Pts',(-1.96514941456394,0.801424913922105,
28.2605650008325));
#23804=CARTESIAN_POINT('Ctrl Pts',(-0.392558968632649,2.08562595723233,
28.149431882841));
#23805=CARTESIAN_POINT('Ctrl Pts',(1.53928926934995,1.46102410423217,28.0382987648494));
#23806=CARTESIAN_POINT('Ctrl Pts',(2.06233375318916,-0.500787438181385,
27.9271656468578));
#23807=CARTESIAN_POINT('Ctrl Pts',(0.697841737943671,-2.00424668184208,
27.8160325288663));
#23808=CARTESIAN_POINT('Ctrl Pts',(-1.30533861404847,-1.67334667879575,
27.7048994108747));
#23809=CARTESIAN_POINT('Ctrl Pts',(-2.11382371160785,0.189069293587439,
27.5937662928831));
#23810=CARTESIAN_POINT('Ctrl Pts',(-0.98765309680873,1.87843992836297,27.4826331748916));
#23811=CARTESIAN_POINT('Ctrl Pts',(1.04245595850156,1.8485892791062,27.3715000569));
#23812=CARTESIAN_POINT('Ctrl Pts',(2.11846857463714,0.126836507687731,27.2603669389085));
#23813=CARTESIAN_POINT('Ctrl Pts',(1.25557522105255,-1.71100179155877,27.1492338209169));
#23814=CARTESIAN_POINT('Ctrl Pts',(-0.756469916759,-1.98286402968576,27.0381007029254));
#23815=CARTESIAN_POINT('Ctrl Pts',(-2.07616405246128,-0.439930999152115,
26.9269675849338));
#23816=CARTESIAN_POINT('Ctrl Pts',(-1.49567110948434,1.50564416406869,26.8158344669423));
#23817=CARTESIAN_POINT('Ctrl Pts',(0.453718891090288,2.07319454405416,26.7047013489507));
#23818=CARTESIAN_POINT('Ctrl Pts',(1.98784750997817,0.743275668181553,26.5935682309591));
#23819=CARTESIAN_POINT('Ctrl Pts',(1.70261984388434,-1.26691834957566,26.4824351129675));
#23820=CARTESIAN_POINT('Ctrl Pts',(-0.140912516270202,-2.11757883081554,
26.371301994976));
#23821=CARTESIAN_POINT('Ctrl Pts',(-1.85547619606559,-1.03014781773599,
26.2601688769844));
#23822=CARTESIAN_POINT('Ctrl Pts',(-1.87183502997734,1.00011502369975,26.1490357589929));
#23823=CARTESIAN_POINT('Ctrl Pts',(-0.175016769959812,2.11503323164442,
26.0379026410014));
#23824=CARTESIAN_POINT('Ctrl Pts',(1.68198372662962,1.29418977891308,25.9267695230097));
#23825=CARTESIAN_POINT('Ctrl Pts',(1.99956651431514,-0.711147098200105,
25.8156364050183));
#23826=CARTESIAN_POINT('Ctrl Pts',(0.4870673259586,-2.06561416061176,25.7045032870266));
#23827=CARTESIAN_POINT('Ctrl Pts',(-1.47121504991412,-1.52954984142534,
25.5933701690351));
#23828=CARTESIAN_POINT('Ctrl Pts',(-2.08298350563717,0.406418695115622,
25.4822370510435));
#23829=CARTESIAN_POINT('Ctrl Pts',(-0.788323471573461,1.97041684540958,
25.371103933052));
#23830=CARTESIAN_POINT('Ctrl Pts',(1.22784123178597,1.73101194392987,25.2599708150604));
#23831=CARTESIAN_POINT('Ctrl Pts',(2.12023731245378,-0.0926832205988131,
25.1488376970689));
#23832=CARTESIAN_POINT('Ctrl Pts',(1.07210875303708,-1.83155105366041,25.0377045790773));
#23833=CARTESIAN_POINT('Ctrl Pts',(-0.957255934948788,-1.89411127326451,
24.9265714610857));
#23834=CARTESIAN_POINT('Ctrl Pts',(-2.11050231404291,-0.223106304083948,
24.8154383430942));
#23835=CARTESIAN_POINT('Ctrl Pts',(-1.33213390676344,1.65209433597293,24.7043052251026));
#23836=CARTESIAN_POINT('Ctrl Pts',(0.665455884265618,2.0152332139479,24.5931721071111));
#23837=CARTESIAN_POINT('Ctrl Pts',(2.05399425792638,0.533951335711417,24.4820389891195));
#23838=CARTESIAN_POINT('Ctrl Pts',(1.56263624230674,-1.43602382108795,24.370905871128));
#23839=CARTESIAN_POINT('Ctrl Pts',(-0.358907967035191,-2.09169345548081,
24.2597727531364));
#23840=CARTESIAN_POINT('Ctrl Pts',(-1.95196547846659,-0.832962911165477,
24.1486396351448));
#23841=CARTESIAN_POINT('Ctrl Pts',(-1.75850735539279,1.1881280745492,24.0375065171533));
#23842=CARTESIAN_POINT('Ctrl Pts',(0.0444059135115228,2.12179748217114,
23.9263733991617));
#23843=CARTESIAN_POINT('Ctrl Pts',(1.80667714257038,1.11351432097495,23.8152402811702));
#23844=CARTESIAN_POINT('Ctrl Pts',(1.91540634062942,-0.9139009742741,23.7041071631786));
#23845=CARTESIAN_POINT('Ctrl Pts',(0.271080266085507,-2.10487812707567,
23.592974045187));
#23846=CARTESIAN_POINT('Ctrl Pts',(-1.62134913759518,-1.36938797078182,
23.4818409271955));
#23847=CARTESIAN_POINT('Ctrl Pts',(-2.02985599486855,0.619419954956861,
23.3707078092039));
#23848=CARTESIAN_POINT('Ctrl Pts',(-0.580558751284808,2.04131035778717,
23.2595746912124));
#23849=CARTESIAN_POINT('Ctrl Pts',(1.40008871204456,1.59491317597791,23.1484415732208));
#23850=CARTESIAN_POINT('Ctrl Pts',(2.09931987915605,-0.311211319657211,
23.0373084552292));
#23851=CARTESIAN_POINT('Ctrl Pts',(0.87717086443866,-1.93250296638388,22.9261753372377));
#23852=CARTESIAN_POINT('Ctrl Pts',(-1.14779945052178,-1.78509183570046,
22.8150422192461));
#23853=CARTESIAN_POINT('Ctrl Pts',(-2.12225853141856,-0.00389439645398614,
22.7039091012546));
#23854=CARTESIAN_POINT('Ctrl Pts',(-1.15434307307923,1.78086734770913,22.592775983263));
#23855=CARTESIAN_POINT('Ctrl Pts',(0.870072600242795,1.93570920099308,22.4816428652714));
#23856=CARTESIAN_POINT('Ctrl Pts',(2.09816358409882,0.318913804756463,22.3705097472799));
#23857=CARTESIAN_POINT('Ctrl Pts',(1.4059326728736,-1.58976405791833,22.2593766292883));
#23858=CARTESIAN_POINT('Ctrl Pts',(-0.573063157536151,-2.04342728228266,
22.1482435112968));
#23859=CARTESIAN_POINT('Ctrl Pts',(-2.02756903062303,-0.62686542938788,
22.0371103933052));
#23860=CARTESIAN_POINT('Ctrl Pts',(-1.62636392254376,1.3634283376657,21.9259772753137));
#23861=CARTESIAN_POINT('Ctrl Pts',(0.263353460506672,2.1058588260709,21.8148441573221));
#23862=CARTESIAN_POINT('Ctrl Pts',(1.9120393910123,0.920924431060889,21.7037110393305));
#23863=CARTESIAN_POINT('Ctrl Pts',(1.81075161372237,-1.10687625048956,21.592577921339));
#23864=CARTESIAN_POINT('Ctrl Pts',(0.052192689072424,-2.12162022136514,
21.4814448033474));
#23865=CARTESIAN_POINT('Ctrl Pts',(-1.75413503891566,-1.19457385949326,
21.3703116853558));
#23866=CARTESIAN_POINT('Ctrl Pts',(-1.95500933717726,0.825793516563662,
21.2591785673643));
#23867=CARTESIAN_POINT('Ctrl Pts',(-0.366582141691425,2.09036216333028,
21.1480454493727));
#23868=CARTESIAN_POINT('Ctrl Pts',(1.55735545850838,1.44174908239318,21.0369123313812));
#23869=CARTESIAN_POINT('Ctrl Pts',(2.055940045965,-0.526409505497094,20.9257792133896));
#23870=CARTESIAN_POINT('Ctrl Pts',(0.672847382732627,-2.01277739457252,
20.814646095398));
#23871=CARTESIAN_POINT('Ctrl Pts',(-1.32606168894103,-1.65697219019589,
20.7035129774065));
#23872=CARTESIAN_POINT('Ctrl Pts',(-2.11130690817558,0.215359180835817,
20.5923798594149));
#23873=CARTESIAN_POINT('Ctrl Pts',(-0.964200947587525,1.89058535234685,
20.4812467414234));
#23874=CARTESIAN_POINT('Ctrl Pts',(1.06537967613682,1.8354733981463,20.3701136234318));
#23875=CARTESIAN_POINT('Ctrl Pts',(2.11988287708905,0.100463943606212,20.2589805054403));
#23876=CARTESIAN_POINT('Ctrl Pts',(1.23418585083075,-1.72649406090975,20.1478473874487));
#23877=CARTESIAN_POINT('Ctrl Pts',(-0.781086681019479,-1.97329675718504,
20.0367142694571));
#23878=CARTESIAN_POINT('Ctrl Pts',(-2.08147786640381,-0.414060572995714,
19.9255811514656));
#23879=CARTESIAN_POINT('Ctrl Pts',(-1.47681872209176,1.52414010625231,19.814448033474));
#23880=CARTESIAN_POINT('Ctrl Pts',(0.479483312463692,2.06738784491702,19.7033149154825));
#23881=CARTESIAN_POINT('Ctrl Pts',(1.99694283049276,0.718480713622634,19.5921817974909));
#23882=CARTESIAN_POINT('Ctrl Pts',(1.68672266442399,-1.28800797157924,19.4810486794994));
#23883=CARTESIAN_POINT('Ctrl Pts',(-0.167254382363781,-2.11566159305851,
19.3699155615078));
#23884=CARTESIAN_POINT('Ctrl Pts',(-1.86814996453264,-1.0069774391256,19.2587824435162));
#23885=CARTESIAN_POINT('Ctrl Pts',(-1.85924822631064,1.0233301523674,19.1476493255247));
#23886=CARTESIAN_POINT('Ctrl Pts',(-0.148675765957402,2.11704945726364,
19.0365162075331));
#23887=CARTESIAN_POINT('Ctrl Pts',(1.69794452754165,1.27315456984867,18.9253830895415));
#23888=CARTESIAN_POINT('Ctrl Pts',(1.99058929493877,-0.735967644051852,
18.81424997155));
#23889=CARTESIAN_POINT('Ctrl Pts',(0.461272008464836,-2.07152992199117,
18.7031168535584));
#23890=CARTESIAN_POINT('Ctrl Pts',(-1.49003428616897,-1.51109530584743,
18.5919837355669));
#23891=CARTESIAN_POINT('Ctrl Pts',(-2.07795878442334,0.43225481623207,18.4808506175753));
#23892=CARTESIAN_POINT('Ctrl Pts',(-0.763368548172731,1.9801776096923,18.3697174995837));
#23893=CARTESIAN_POINT('Ctrl Pts',(1.24856735077038,1.71539873057631,18.2585843815922));
#23894=CARTESIAN_POINT('Ctrl Pts',(2.12032280000797,-0.118666593922666,
18.1474512636006));
#23895=CARTESIAN_POINT('Ctrl Pts',(1.04636073931038,-1.84560680034591,18.0363181456091));
#23896=CARTESIAN_POINT('Ctrl Pts',(-0.300314735083234,-1.86826056061615,
17.9622294002814));
#23897=CARTESIAN_POINT('Ctrl Pts',(-0.829785877867478,-1.59234886373437,
17.9251850276175));
#23898=CARTESIAN_POINT('Ctrl Pts',(-0.429864256885881,-1.60958774866484,
29.2244449171475));
#23899=CARTESIAN_POINT('Ctrl Pts',(-0.965067492876795,-1.46665379460549,
29.1874005444836));
#23900=CARTESIAN_POINT('Ctrl Pts',(-1.87243069143824,-0.607377246303806,
29.1133117991559));
#23901=CARTESIAN_POINT('Ctrl Pts',(-1.52533145026359,1.24730530523812,29.0021786811643));
#23902=CARTESIAN_POINT('Ctrl Pts',(0.220381886651061,1.95618532526583,28.8910455631728));
#23903=CARTESIAN_POINT('Ctrl Pts',(1.76309023385211,0.876778588782393,28.7799124451812));
#23904=CARTESIAN_POINT('Ctrl Pts',(1.69282300260543,-1.00616693362718,28.6687793271896));
#23905=CARTESIAN_POINT('Ctrl Pts',(0.0728673284468312,-1.96767010293874,
28.5576462091981));
#23906=CARTESIAN_POINT('Ctrl Pts',(-1.61359726760772,-1.12857467982718,
28.4465130912066));
#23907=CARTESIAN_POINT('Ctrl Pts',(-1.82332886694028,0.743587825643046,
28.335379973215));
#23908=CARTESIAN_POINT('Ctrl Pts',(-0.364228843964538,1.93511088026123,
28.2242468552234));
#23909=CARTESIAN_POINT('Ctrl Pts',(1.4282021196846,1.3555851808516,28.1131137372319));
#23910=CARTESIAN_POINT('Ctrl Pts',(1.91349962378789,-0.464646700892107,
28.0019806192403));
#23911=CARTESIAN_POINT('Ctrl Pts',(0.647480021579331,-1.85960456970283,
27.8908475012488));
#23912=CARTESIAN_POINT('Ctrl Pts',(-1.21113517297336,-1.55258489824498,
27.7797143832572));
#23913=CARTESIAN_POINT('Ctrl Pts',(-1.96127366419753,0.175424574994203,
27.6685812652656));
#23914=CARTESIAN_POINT('Ctrl Pts',(-0.916376326699777,1.74287701526117,
27.5574481472741));
#23915=CARTESIAN_POINT('Ctrl Pts',(0.967224185379086,1.71518062226255,27.4463150292825));
#23916=CARTESIAN_POINT('Ctrl Pts',(1.96558331759158,0.117682993534743,27.335181911291));
#23917=CARTESIAN_POINT('Ctrl Pts',(1.16496309552525,-1.58752252363869,27.2240487932994));
#23918=CARTESIAN_POINT('Ctrl Pts',(-0.701877132586712,-1.83976505692104,
27.1129156753079));
#23919=CARTESIAN_POINT('Ctrl Pts',(-1.92633182052286,-0.408182138351005,
27.0017825573162));
#23920=CARTESIAN_POINT('Ctrl Pts',(-1.3877317872934,1.39698510827778,26.8906494393248));
#23921=CARTESIAN_POINT('Ctrl Pts',(0.420974988196826,1.92357661506153,26.7795163213331));
#23922=CARTESIAN_POINT('Ctrl Pts',(1.8443888903088,0.689635084154899,26.6683832033416));
#23923=CARTESIAN_POINT('Ctrl Pts',(1.57974548284846,-1.1754876152001,26.55725008535));
#23924=CARTESIAN_POINT('Ctrl Pts',(-0.130743167274974,-1.96475778464122,
26.4461169673585));
#23925=CARTESIAN_POINT('Ctrl Pts',(-1.72157052544407,-0.955804296290804,
26.3349838493669));
#23926=CARTESIAN_POINT('Ctrl Pts',(-1.73674877798798,0.927938903504224,
26.2238507313754));
#23927=CARTESIAN_POINT('Ctrl Pts',(-0.16238619135084,1.9623958958108,26.1127176133838));
#23928=CARTESIAN_POINT('Ctrl Pts',(1.56059862917248,1.20079092495615,26.0015844953923));
#23929=CARTESIAN_POINT('Ctrl Pts',(1.85526215965974,-0.659825163002576,
25.8904513774007));
#23930=CARTESIAN_POINT('Ctrl Pts',(0.451916739247426,-1.91654329136076,
25.7793182594092));
#23931=CARTESIAN_POINT('Ctrl Pts',(-1.36504066820824,-1.41916556503343,
25.6681851414176));
#23932=CARTESIAN_POINT('Ctrl Pts',(-1.93265912863499,0.377088344212721,
25.557052023426));
#23933=CARTESIAN_POINT('Ctrl Pts',(-0.731431885816894,1.82821615878909,
25.4459189054345));
#23934=CARTESIAN_POINT('Ctrl Pts',(1.13923060778136,1.60608858695159,25.3347857874429));
#23935=CARTESIAN_POINT('Ctrl Pts',(1.96722440945728,-0.0859944746930651,
25.2236526694514));
#23936=CARTESIAN_POINT('Ctrl Pts',(0.994737002400207,-1.69937200838998,
25.1125195514598));
#23937=CARTESIAN_POINT('Ctrl Pts',(-0.88817286172071,-1.75741739337746,
25.0013864334682));
#23938=CARTESIAN_POINT('Ctrl Pts',(-1.9581919646515,-0.207005208671568,
24.8902533154767));
#23939=CARTESIAN_POINT('Ctrl Pts',(-1.23599670784864,1.53286629065628,24.7791201974851));
#23940=CARTESIAN_POINT('Ctrl Pts',(0.6174313843337,1.86979822774616,24.6679870794936));
#23941=CARTESIAN_POINT('Ctrl Pts',(1.90576197171134,0.495417232261691,24.556853961502));
#23942=CARTESIAN_POINT('Ctrl Pts',(1.44986419251851,-1.33238911362094,24.4457208435104));
#23943=CARTESIAN_POINT('Ctrl Pts',(-0.333006361765792,-1.9407405003932,
24.3345877255189));
#23944=CARTESIAN_POINT('Ctrl Pts',(-1.81109638675937,-0.772849794403871,
24.2234546075273));
#23945=CARTESIAN_POINT('Ctrl Pts',(-1.63159971453162,1.10238346249536,24.1123214895358));
#23946=CARTESIAN_POINT('Ctrl Pts',(0.0412012355744378,1.96867198512857,
24.0011883715442));
#23947=CARTESIAN_POINT('Ctrl Pts',(1.67629319321794,1.03315442079785,23.8900552535526));
#23948=CARTESIAN_POINT('Ctrl Pts',(1.77717564217123,-0.847946734008808,
23.7789221355611));
#23949=CARTESIAN_POINT('Ctrl Pts',(0.251516994457764,-1.95297366299238,
23.6677890175695));
#23950=CARTESIAN_POINT('Ctrl Pts',(-1.50433990619589,-1.270562227311,23.556655899578));
#23951=CARTESIAN_POINT('Ctrl Pts',(-1.88336571445733,0.574717767647355,
23.4455227815863));
#23952=CARTESIAN_POINT('Ctrl Pts',(-0.538661092295258,1.89399344098395,
23.3343896635949));
#23953=CARTESIAN_POINT('Ctrl Pts',(1.29904736302942,1.47981177027663,23.2232565456032));
#23954=CARTESIAN_POINT('Ctrl Pts',(1.94781654170361,-0.288751877411564,
23.1121234276117));
#23955=CARTESIAN_POINT('Ctrl Pts',(0.813867356098656,-1.79303844172955,
23.0009903096202));
#23956=CARTESIAN_POINT('Ctrl Pts',(-1.06496526731478,-1.65626565087129,
22.8898571916286));
#23957=CARTESIAN_POINT('Ctrl Pts',(-1.96909976145727,-0.00361334635485625,
22.778724073637));
#23958=CARTESIAN_POINT('Ctrl Pts',(-1.07103665090268,1.65234603496547,22.6675909556455));
#23959=CARTESIAN_POINT('Ctrl Pts',(0.807281358149812,1.7960132893792,22.5564578376539));
#23960=CARTESIAN_POINT('Ctrl Pts',(1.946743693939,0.295898490958891,22.4453247196624));
#23961=CARTESIAN_POINT('Ctrl Pts',(1.30446957795002,-1.47503425283813,22.3341916016708));
#23962=CARTESIAN_POINT('Ctrl Pts',(-0.531706439200944,-1.89595759165521,
22.2230584836793));
#23963=CARTESIAN_POINT('Ctrl Pts',(-1.88124379543396,-0.581625918425882,
22.1119253656877));
#23964=CARTESIAN_POINT('Ctrl Pts',(-1.50899278505104,1.26503268792002,22.0007922476961));
#23965=CARTESIAN_POINT('Ctrl Pts',(0.244347815586829,1.95388358707985,21.8896591297046));
#23966=CARTESIAN_POINT('Ctrl Pts',(1.77405167796528,0.854463323236147,21.778526011713));
#23967=CARTESIAN_POINT('Ctrl Pts',(1.68007361867256,-1.02699540538299,21.6673928937215));
#23968=CARTESIAN_POINT('Ctrl Pts',(0.0484260565246162,-1.96850751684837,
21.5562597757299));
#23969=CARTESIAN_POINT('Ctrl Pts',(-1.62754293859943,-1.10836406919707,
21.4451266577384));
#23970=CARTESIAN_POINT('Ctrl Pts',(-1.81392057682497,0.766197799375352,
21.3339935397467));
#23971=CARTESIAN_POINT('Ctrl Pts',(-0.340126707973034,1.93950528469388,
21.2228604217553));
#23972=CARTESIAN_POINT('Ctrl Pts',(1.44496451137047,1.33770119530349,21.1117273037636));
#23973=CARTESIAN_POINT('Ctrl Pts',(1.90756733647061,-0.488419679486605,
21.0005941857721));
#23974=CARTESIAN_POINT('Ctrl Pts',(0.624289454475828,-1.86751963949941,
20.8894610677805));
#23975=CARTESIAN_POINT('Ctrl Pts',(-1.2303627087441,-1.53739212077766,20.778327949789));
#23976=CARTESIAN_POINT('Ctrl Pts',(-1.95893849298029,0.19981717841322,20.6671948317974));
#23977=CARTESIAN_POINT('Ctrl Pts',(-0.894616667943091,1.75414593048305,
20.5560617138059));
#23978=CARTESIAN_POINT('Ctrl Pts',(0.988493548304972,1.70301128582823,20.4449285958143));
#23979=CARTESIAN_POINT('Ctrl Pts',(1.96689555291986,0.0932136798893295,
20.3337954778228));
#23980=CARTESIAN_POINT('Ctrl Pts',(1.14511734950612,-1.60189674969638,20.2226623598312));
#23981=CARTESIAN_POINT('Ctrl Pts',(-0.7247173586551,-1.83088823361226,20.1115292418396));
#23982=CARTESIAN_POINT('Ctrl Pts',(-1.93126214810159,-0.384178724431723,
20.0003961238481));
#23983=CARTESIAN_POINT('Ctrl Pts',(-1.37023993558539,1.41414623865022,19.8892630058565));
#23984=CARTESIAN_POINT('Ctrl Pts',(0.444880047467124,1.91818897273778,19.778129887865));
#23985=CARTESIAN_POINT('Ctrl Pts',(1.85282782137705,0.666629527393313,19.6669967698734));
#23986=CARTESIAN_POINT('Ctrl Pts',(1.56499556816097,-1.19505524517623,19.5558636518819));
#23987=CARTESIAN_POINT('Ctrl Pts',(-0.15518399833929,-1.96297890975197,
19.4447305338902));
#23988=CARTESIAN_POINT('Ctrl Pts',(-1.73332965567998,-0.934306073374439,
19.3335974158987));
#23989=CARTESIAN_POINT('Ctrl Pts',(-1.72507033649243,0.949478646963803,
19.2224642979071));
#23990=CARTESIAN_POINT('Ctrl Pts',(-0.137946160162454,1.96426661482409,
19.1113311799156));
#23991=CARTESIAN_POINT('Ctrl Pts',(1.57540757389023,1.18127378105604,19.000198061924));
#23992=CARTESIAN_POINT('Ctrl Pts',(1.8469328066281,-0.682854464189196,18.8890649439325));
#23993=CARTESIAN_POINT('Ctrl Pts',(0.427983013562401,-1.9220321251426,18.7779318259409));
#23994=CARTESIAN_POINT('Ctrl Pts',(-1.38250176122384,-1.40204285304227,
18.6667987079494));
#23995=CARTESIAN_POINT('Ctrl Pts',(-1.92799703059319,0.401059928811971,
18.5556655899578));
#23996=CARTESIAN_POINT('Ctrl Pts',(-0.708277904815949,1.83727250999993,
18.4445324719662));
#23997=CARTESIAN_POINT('Ctrl Pts',(1.15846096795848,1.59160214515625,18.3333993539747));
#23998=CARTESIAN_POINT('Ctrl Pts',(1.96730372756111,-0.110102684629042,
18.2222662359831));
#23999=CARTESIAN_POINT('Ctrl Pts',(0.97084716667254,-1.71241338249015,18.1111331179916));
#24000=CARTESIAN_POINT('Ctrl Pts',(-0.278641675582867,-1.73343227028533,
18.0370443726639));
#24001=CARTESIAN_POINT('Ctrl Pts',(-0.76990204067047,-1.47743251885541,
18.));
#24002=CARTESIAN_POINT('Ctrl Pts',(-1.6638200260918,0.000942871389988137,
28.3785196366098));
#24003=CARTESIAN_POINT('Ctrl Pts',(-1.66493926816573,0.216633787367396,
28.3641397488115));
#24004=CARTESIAN_POINT('Ctrl Pts',(-1.62602025375689,0.431937629364058,
28.3497598610133));
#24005=CARTESIAN_POINT('Ctrl Pts',(-1.54519026322223,0.630147917167703,
28.335379973215));
#24006=CARTESIAN_POINT('Ctrl Pts',(-1.33696219261504,1.14076217718244,28.2983356005511));
#24007=CARTESIAN_POINT('Ctrl Pts',(-0.850595518289787,1.53793652872184,
28.2612912278873));
#24008=CARTESIAN_POINT('Ctrl Pts',(-0.308673687185639,1.63993608792326,
28.2242468552234));
#24009=CARTESIAN_POINT('Ctrl Pts',(0.23324814391851,1.74193564712469,28.1872024825596));
#24010=CARTESIAN_POINT('Ctrl Pts',(0.830725131801557,1.54876041398814,28.1501581098957));
#24011=CARTESIAN_POINT('Ctrl Pts',(1.21034654309363,1.14880081712925,28.1131137372319));
#24012=CARTESIAN_POINT('Ctrl Pts',(1.5899679543857,0.748841220270365,28.076069364568));
#24013=CARTESIAN_POINT('Ctrl Pts',(1.75173378908679,0.142097259689129,28.0390249919042));
#24014=CARTESIAN_POINT('Ctrl Pts',(1.62161343940258,-0.393767698736607,
28.0019806192403));
#24015=CARTESIAN_POINT('Ctrl Pts',(1.49149308971837,-0.929632657162347,
27.9649362465765));
#24016=CARTESIAN_POINT('Ctrl Pts',(1.06948655564886,-1.39461861343258,27.9278918739126));
#24017=CARTESIAN_POINT('Ctrl Pts',(0.548714089521982,-1.57594164632473,
27.8908475012488));
#24018=CARTESIAN_POINT('Ctrl Pts',(0.0279416233951079,-1.75726467921688,
27.8538031285849));
#24019=CARTESIAN_POINT('Ctrl Pts',(-0.591596774789128,-1.65492478873093,
27.8167587559211));
#24020=CARTESIAN_POINT('Ctrl Pts',(-1.02638905575194,-1.31575326461476,
27.7797143832572));
#24021=CARTESIAN_POINT('Ctrl Pts',(-1.42229889353421,-1.00691304602614,
27.7459828010414));
#24022=CARTESIAN_POINT('Ctrl Pts',(-1.66502795857797,-0.501705763306371,
27.7122512188256));
#24023=CARTESIAN_POINT('Ctrl Pts',(-1.66818493320164,0.000858898907110364,
27.6785196366098));
#24024=CARTESIAN_POINT('Ctrl Pts',(-0.530170217188634,-1.98517432567172,
29.));
#24025=CARTESIAN_POINT('Ctrl Pts',(-0.598844984340848,-1.9597466054765,
29.));
#24026=CARTESIAN_POINT('Ctrl Pts',(-0.665816349367419,-1.93043078959701,
29.));
#24027=CARTESIAN_POINT('Ctrl Pts',(-0.730895187105961,-1.8975204208506,
29.));
#24028=CARTESIAN_POINT('Ctrl Pts',(-0.797776356373901,-1.86369861303587,
29.));
#24029=CARTESIAN_POINT('Ctrl Pts',(-0.862659492565893,-1.82607970767592,
29.));
#24030=CARTESIAN_POINT('Ctrl Pts',(-0.925308102267728,-1.78493769378496,
29.));
#24031=CARTESIAN_POINT('Ctrl Pts',(-0.978240206862307,-1.75017661300644,
29.));
#24032=CARTESIAN_POINT('Ctrl Pts',(-1.02957682932671,-1.71289946201033,
29.));
#24033=CARTESIAN_POINT('Ctrl Pts',(-1.07915259076278,-1.67325348841043,
29.));
#24034=CARTESIAN_POINT('Ctrl Pts',(-1.10117709167781,-1.65564038965945,
29.));
#24035=CARTESIAN_POINT('Ctrl Pts',(-1.12285375455339,-1.63755958589035,
29.));
#24036=CARTESIAN_POINT('Ctrl Pts',(-1.14416652638477,-1.61902326437413,
29.));
#24037=CARTESIAN_POINT('Ctrl Pts',(-1.15588198328982,-1.60883399956992,
29.));
#24038=CARTESIAN_POINT('Ctrl Pts',(-1.16748746879726,-1.59850708840077,
29.));
#24039=CARTESIAN_POINT('Ctrl Pts',(-1.17898018224506,-1.58804451337869,
29.));
#24040=CARTESIAN_POINT('Ctrl Pts',(-1.18957053268403,-1.57840341891643,
29.));
#24041=CARTESIAN_POINT('Ctrl Pts',(-1.20006655223653,-1.56864561876181,
29.));
#24042=CARTESIAN_POINT('Ctrl Pts',(-1.21045017554235,-1.55878810261091,
29.));
#24043=CARTESIAN_POINT('Ctrl Pts',(-1.26353644073431,-1.50839155979456,
29.));
#24044=CARTESIAN_POINT('Ctrl Pts',(-1.31378278231012,-1.45530711011964,
29.));
#24045=CARTESIAN_POINT('Ctrl Pts',(-1.36097043055599,-1.3997936077315,29.));
#24046=CARTESIAN_POINT('Ctrl Pts',(-1.40778995980368,-1.34471317576845,
29.));
#24047=CARTESIAN_POINT('Ctrl Pts',(-1.45159884056718,-1.28724056013132,
29.));
#24048=CARTESIAN_POINT('Ctrl Pts',(-1.4921385971107,-1.22760436053223,29.));
#24049=CARTESIAN_POINT('Ctrl Pts',(-1.5258287787978,-1.17804426025226,29.));
#24050=CARTESIAN_POINT('Ctrl Pts',(-1.55726056691569,-1.12698927604103,
29.));
#24051=CARTESIAN_POINT('Ctrl Pts',(-1.58625800648523,-1.07456412141552,
29.));
#24052=CARTESIAN_POINT('Ctrl Pts',(-1.59836554642316,-1.052674614521,29.));
#24053=CARTESIAN_POINT('Ctrl Pts',(-1.6100483646418,-1.03054619530609,29.));
#24054=CARTESIAN_POINT('Ctrl Pts',(-1.62129221084824,-1.00818785804745,
29.));
#24055=CARTESIAN_POINT('Ctrl Pts',(-1.62649432232627,-0.997843482933499,
29.));
#24056=CARTESIAN_POINT('Ctrl Pts',(-1.63160245634821,-0.987449892279893,
29.));
#24057=CARTESIAN_POINT('Ctrl Pts',(-1.63661513633768,-0.977007978776379,
29.));
#24058=CARTESIAN_POINT('Ctrl Pts',(-1.64184640941963,-0.96611071400989,
29.));
#24059=CARTESIAN_POINT('Ctrl Pts',(-1.64697010952128,-0.955168277699256,
29.));
#24060=CARTESIAN_POINT('Ctrl Pts',(-1.6519831845252,-0.944185960007519,
29.));
#24061=CARTESIAN_POINT('Ctrl Pts',(-1.68052299443904,-0.881662806236541,
29.));
#24062=CARTESIAN_POINT('Ctrl Pts',(-1.70550187231934,-0.817805134572764,
29.));
#24063=CARTESIAN_POINT('Ctrl Pts',(-1.72669629748412,-0.752816828589081,
29.));
#24064=CARTESIAN_POINT('Ctrl Pts',(-1.74589987179783,-0.693933053550302,
29.));
#24065=CARTESIAN_POINT('Ctrl Pts',(-1.76199624844007,-0.634120477883048,
29.));
#24066=CARTESIAN_POINT('Ctrl Pts',(-1.77478245715023,-0.573525911714975,
29.));
#24067=CARTESIAN_POINT('Ctrl Pts',(-1.78991431693715,-0.501815172441987,
29.));
#24068=CARTESIAN_POINT('Ctrl Pts',(-1.80041069773216,-0.42900768942451,
29.));
#24069=CARTESIAN_POINT('Ctrl Pts',(-1.80634685634798,-0.355527190631044,
29.));
#24070=CARTESIAN_POINT('Ctrl Pts',(-1.80765324390704,-0.339356125187838,
29.));
#24071=CARTESIAN_POINT('Ctrl Pts',(-1.80873854664514,-0.323152545934638,
29.));
#24072=CARTESIAN_POINT('Ctrl Pts',(-1.80960319748954,-0.306921133556182,
29.));
#24073=CARTESIAN_POINT('Ctrl Pts',(-1.81049819138598,-0.290120114852003,
29.));
#24074=CARTESIAN_POINT('Ctrl Pts',(-1.81115678487511,-0.27328307874498,
29.));
#24075=CARTESIAN_POINT('Ctrl Pts',(-1.81157889796795,-0.256449498362707,
29.));
#24076=CARTESIAN_POINT('Ctrl Pts',(-1.81329830981387,-0.18788053424027,
29.));
#24077=CARTESIAN_POINT('Ctrl Pts',(-1.81110575709439,-0.119282211213726,
29.));
#24078=CARTESIAN_POINT('Ctrl Pts',(-1.80512192796928,-0.0509934048330952,
29.));
#24079=CARTESIAN_POINT('Ctrl Pts',(-1.79913941487413,0.0172803827172064,
29.));
#24080=CARTESIAN_POINT('Ctrl Pts',(-1.78936683881028,0.0852458626519091,
29.));
#24081=CARTESIAN_POINT('Ctrl Pts',(-1.77587520290159,0.152549360262613,
29.));
#24082=CARTESIAN_POINT('Ctrl Pts',(-1.76611529025284,0.2012370258712,29.));
#24083=CARTESIAN_POINT('Ctrl Pts',(-1.75440809028966,0.249578001150906,
29.));
#24084=CARTESIAN_POINT('Ctrl Pts',(-1.74076629009681,0.297428750832602,
29.));
#24085=CARTESIAN_POINT('Ctrl Pts',(-1.73053117355718,0.333330024313932,
29.));
#24086=CARTESIAN_POINT('Ctrl Pts',(-1.71920679407154,0.368955188045359,
29.));
#24087=CARTESIAN_POINT('Ctrl Pts',(-1.70679459856354,0.404239446148925,
29.));
#24088=CARTESIAN_POINT('Ctrl Pts',(-1.70266053149517,0.415991395218995,
29.));
#24089=CARTESIAN_POINT('Ctrl Pts',(-1.69840897216887,0.427696366036902,
29.));
#24090=CARTESIAN_POINT('Ctrl Pts',(-1.69404059684701,0.439351704919061,
29.));
#24091=CARTESIAN_POINT('Ctrl Pts',(-1.67091592294313,0.501051053310776,
29.));
#24092=CARTESIAN_POINT('Ctrl Pts',(-1.64451911211263,0.561366930679729,
29.));
#24093=CARTESIAN_POINT('Ctrl Pts',(-1.61490024705089,0.619964816031714,
29.));
#24094=CARTESIAN_POINT('Ctrl Pts',(-1.5940694639762,0.661176382911764,29.));
#24095=CARTESIAN_POINT('Ctrl Pts',(-1.57164412390922,0.701537662145848,
29.));
#24096=CARTESIAN_POINT('Ctrl Pts',(-1.5476312537223,0.740920937772863,29.));
#24097=CARTESIAN_POINT('Ctrl Pts',(-1.53991733315498,0.75357246412114,29.));
#24098=CARTESIAN_POINT('Ctrl Pts',(-1.53203843675107,0.766124659274376,
29.));
#24099=CARTESIAN_POINT('Ctrl Pts',(-1.52399809481428,0.778567695014452,
29.));
#24100=CARTESIAN_POINT('Ctrl Pts',(-1.48975623557589,0.831559555517324,
29.));
#24101=CARTESIAN_POINT('Ctrl Pts',(-1.45265940234734,0.882467052899552,
29.));
#24102=CARTESIAN_POINT('Ctrl Pts',(-1.4127419174334,0.930974609595389,29.));
#24103=CARTESIAN_POINT('Ctrl Pts',(-1.37594260255018,0.975692979425408,
29.));
#24104=CARTESIAN_POINT('Ctrl Pts',(-1.33674551146281,1.0183718057298,29.));
#24105=CARTESIAN_POINT('Ctrl Pts',(-1.29515607471415,1.05873088388067,29.));
#24106=CARTESIAN_POINT('Ctrl Pts',(-1.28733756798151,1.06631809229016,29.));
#24107=CARTESIAN_POINT('Ctrl Pts',(-1.27943445976865,1.07382321453206,29.));
#24108=CARTESIAN_POINT('Ctrl Pts',(-1.27144834193523,1.08124558643406,29.));
#24109=CARTESIAN_POINT('Origin',(0.,0.,23.));
#24110=CARTESIAN_POINT('Origin',(0.,0.,17.));
#24111=CARTESIAN_POINT('Origin',(6.,-1.,-2.));
#24112=CARTESIAN_POINT('',(-6.,-1.,-2.));
#24113=CARTESIAN_POINT('',(6.,-1.,-2.));
#24114=CARTESIAN_POINT('',(-6.,-1.,-2.));
#24115=CARTESIAN_POINT('',(6.,-1.,-5.));
#24116=CARTESIAN_POINT('',(6.,-1.,-2.));
#24117=CARTESIAN_POINT('',(-6.,-1.,-5.));
#24118=CARTESIAN_POINT('',(3.,-1.,-5.));
#24119=CARTESIAN_POINT('',(-6.,-1.,-2.));
#24120=CARTESIAN_POINT('Origin',(6.,1.,-2.));
#24121=CARTESIAN_POINT('',(6.,1.,-2.));
#24122=CARTESIAN_POINT('',(6.,-1.,-2.));
#24123=CARTESIAN_POINT('',(6.,1.,-5.));
#24124=CARTESIAN_POINT('',(6.,1.,-2.));
#24125=CARTESIAN_POINT('',(6.,0.5,-5.));
#24126=CARTESIAN_POINT('Origin',(-6.,1.,-2.));
#24127=CARTESIAN_POINT('',(-6.,1.,-2.));
#24128=CARTESIAN_POINT('',(6.,1.,-2.));
#24129=CARTESIAN_POINT('',(-6.,1.,-5.));
#24130=CARTESIAN_POINT('',(-6.,1.,-2.));
#24131=CARTESIAN_POINT('',(-3.,1.,-5.));
#24132=CARTESIAN_POINT('Origin',(-6.,-1.,-2.));
#24133=CARTESIAN_POINT('',(-6.,1.,-2.));
#24134=CARTESIAN_POINT('',(-6.,-0.5,-5.));
#24135=CARTESIAN_POINT('Origin',(0.,0.,-2.));
#24136=CARTESIAN_POINT('Origin',(0.,0.,4.));
#24137=CARTESIAN_POINT('',(-3.,-3.67394039744206E-16,3.));
#24138=CARTESIAN_POINT('Origin',(0.,0.,3.));
#24139=CARTESIAN_POINT('',(-3.,-3.67394039744206E-16,5.));
#24140=CARTESIAN_POINT('',(-3.,-3.67394039744206E-16,4.));
#24141=CARTESIAN_POINT('Origin',(0.,0.,5.));
#24142=CARTESIAN_POINT('Origin',(7.,0.,3.));
#24143=CARTESIAN_POINT('',(-4.,4.89858719658941E-16,3.));
#24144=CARTESIAN_POINT('Origin',(0.,0.,3.));
#24145=CARTESIAN_POINT('Origin',(3.,0.,5.));
#24146=CARTESIAN_POINT('',(-4.,-4.89858719658941E-16,5.));
#24147=CARTESIAN_POINT('Origin',(0.,0.,5.));
#24148=CARTESIAN_POINT('Origin',(0.,0.,0.));
#24149=CARTESIAN_POINT('',(-4.,-4.89858719658941E-16,25.));
#24150=CARTESIAN_POINT('Origin',(0.,0.,25.));
#24151=CARTESIAN_POINT('',(-4.,-4.89858719658941E-16,0.));
#24152=CARTESIAN_POINT('Origin',(-1.73205080756888,-3.,25.));
#24153=CARTESIAN_POINT('',(1.73205080756888,-3.,25.));
#24154=CARTESIAN_POINT('',(-1.73205080756888,-3.,25.));
#24155=CARTESIAN_POINT('',(-0.86602540378444,-3.,25.));
#24156=CARTESIAN_POINT('',(1.73205080756888,-3.,29.));
#24157=CARTESIAN_POINT('',(1.73205080756888,-3.,25.));
#24158=CARTESIAN_POINT('',(-1.73205080756888,-3.,29.));
#24159=CARTESIAN_POINT('',(-1.73205080756888,-3.,29.));
#24160=CARTESIAN_POINT('',(-1.73205080756888,-3.,25.));
#24161=CARTESIAN_POINT('Origin',(-3.46410161513775,4.24230095489963E-16,
25.));
#24162=CARTESIAN_POINT('',(-3.46410161513775,4.24230095489963E-16,25.));
#24163=CARTESIAN_POINT('',(-3.03108891324554,-0.749999999999999,25.));
#24164=CARTESIAN_POINT('',(-3.46410161513775,5.55111512312578E-16,29.));
#24165=CARTESIAN_POINT('',(-3.46410161513775,4.24230095489963E-16,29.));
#24166=CARTESIAN_POINT('',(-3.46410161513775,4.24230095489963E-16,25.));
#24167=CARTESIAN_POINT('Origin',(-1.73205080756888,3.,25.));
#24168=CARTESIAN_POINT('',(-1.73205080756888,3.,25.));
#24169=CARTESIAN_POINT('',(-2.1650635094611,2.25,25.));
#24170=CARTESIAN_POINT('',(-1.73205080756888,3.,29.));
#24171=CARTESIAN_POINT('',(-1.73205080756888,3.,29.));
#24172=CARTESIAN_POINT('',(-1.73205080756888,3.,25.));
#24173=CARTESIAN_POINT('Origin',(1.73205080756888,3.,25.));
#24174=CARTESIAN_POINT('',(1.73205080756888,3.,25.));
#24175=CARTESIAN_POINT('',(0.866025403784439,3.,25.));
#24176=CARTESIAN_POINT('',(1.73205080756888,3.,29.));
#24177=CARTESIAN_POINT('',(1.73205080756888,3.,29.));
#24178=CARTESIAN_POINT('',(1.73205080756888,3.,25.));
#24179=CARTESIAN_POINT('Origin',(3.46410161513775,0.,25.));
#24180=CARTESIAN_POINT('',(3.46410161513775,0.,25.));
#24181=CARTESIAN_POINT('',(3.03108891324554,0.75,25.));
#24182=CARTESIAN_POINT('',(3.46410161513775,0.,29.));
#24183=CARTESIAN_POINT('',(3.46410161513775,0.,29.));
#24184=CARTESIAN_POINT('',(3.46410161513775,0.,25.));
#24185=CARTESIAN_POINT('Origin',(1.73205080756888,-3.,25.));
#24186=CARTESIAN_POINT('',(2.1650635094611,-2.25,25.));
#24187=CARTESIAN_POINT('',(1.73205080756888,-3.,29.));
#24188=CARTESIAN_POINT('Origin',(0.,5.55111512312578E-16,29.));
#24189=CARTESIAN_POINT('Origin',(0.,0.,0.));
#24190=CARTESIAN_POINT('',(-10.,-1.22464679914735E-15,0.));
#24191=CARTESIAN_POINT('Origin',(0.,0.,0.));
#24192=CARTESIAN_POINT('',(-4.,-4.89858719658941E-16,0.));
#24193=CARTESIAN_POINT('Origin',(0.,0.,0.));
#24194=CARTESIAN_POINT('Origin',(0.,0.,-5.));
#24195=CARTESIAN_POINT('',(-10.,-1.22464679914735E-15,-5.));
#24196=CARTESIAN_POINT('',(-10.,-1.22464679914735E-15,-5.));
#24197=CARTESIAN_POINT('Origin',(0.,0.,-5.));
#24198=CARTESIAN_POINT('Origin',(0.,0.,-5.));
#24199=CARTESIAN_POINT('Origin',(0.,0.,0.));
#24200=CARTESIAN_POINT('',(-4.,-4.89858719658941E-16,0.));
#24201=CARTESIAN_POINT('Origin',(0.,0.,25.));
#32592=UNCERTAINTY_MEASURE_WITH_UNIT(LENGTH_MEASURE(0.01),#32628,
'DISTANCE_ACCURACY_VALUE',
'Maximum model space distance between geometric entities at asserted c
onnectivities');
#32607=UNCERTAINTY_MEASURE_WITH_UNIT(LENGTH_MEASURE(0.01),#32628,
'DISTANCE_ACCURACY_VALUE',
'Maximum model space distance between geometric entities at asserted c
onnectivities');
#32612=(
GEOMETRIC_REPRESENTATION_CONTEXT(3)
GLOBAL_UNCERTAINTY_ASSIGNED_CONTEXT((#32592))
GLOBAL_UNIT_ASSIGNED_CONTEXT((#32628,#32630,#32631))
REPRESENTATION_CONTEXT('','3D')
);
#32627=(
GEOMETRIC_REPRESENTATION_CONTEXT(3)
GLOBAL_UNCERTAINTY_ASSIGNED_CONTEXT((#32607))
GLOBAL_UNIT_ASSIGNED_CONTEXT((#32628,#32630,#32631))
REPRESENTATION_CONTEXT('','3D')
);
#32628=(
LENGTH_UNIT()
NAMED_UNIT(*)
SI_UNIT(.MILLI.,.METRE.)
);
#32630=(
NAMED_UNIT(*)
PLANE_ANGLE_UNIT()
SI_UNIT($,.RADIAN.)
);
#32631=(
NAMED_UNIT(*)
SI_UNIT($,.STERADIAN.)
SOLID_ANGLE_UNIT()
);
#32636=SHAPE_DEFINITION_REPRESENTATION(#32655,#32711);
#32655=PRODUCT_DEFINITION_SHAPE('',$,#32731);
#32711=SHAPE_REPRESENTATION('',(#9113),#32612);
#32726=PRODUCT_DEFINITION_CONTEXT('part definition',#32785,'design');
#32731=PRODUCT_DEFINITION('Latch spindle','Latch spindle',#32750,#32726);
#32750=PRODUCT_DEFINITION_FORMATION('',$,#32791);
#32785=APPLICATION_CONTEXT(
'Core Data for Automotive Mechanical Design Process');
#32786=PRODUCT_CONTEXT('part definition',#32785,'mechanical');
#32791=PRODUCT('Latch spindle','Latch spindle',$,(#32786));
#32810=PRESENTATION_STYLE_ASSIGNMENT((#32817));
#32817=SURFACE_STYLE_USAGE(.BOTH.,#32824);
#32824=SURFACE_SIDE_STYLE('',(#32831));
#32831=SURFACE_STYLE_FILL_AREA(#32838);
#32838=FILL_AREA_STYLE('Gray',(#32845));
#32845=FILL_AREA_STYLE_COLOUR('Gray',#32852);
#32852=COLOUR_RGB('Gray',0.407843137254902,0.447058823529412,0.498039215686275);
ENDSEC;
END-ISO-10303-21;
